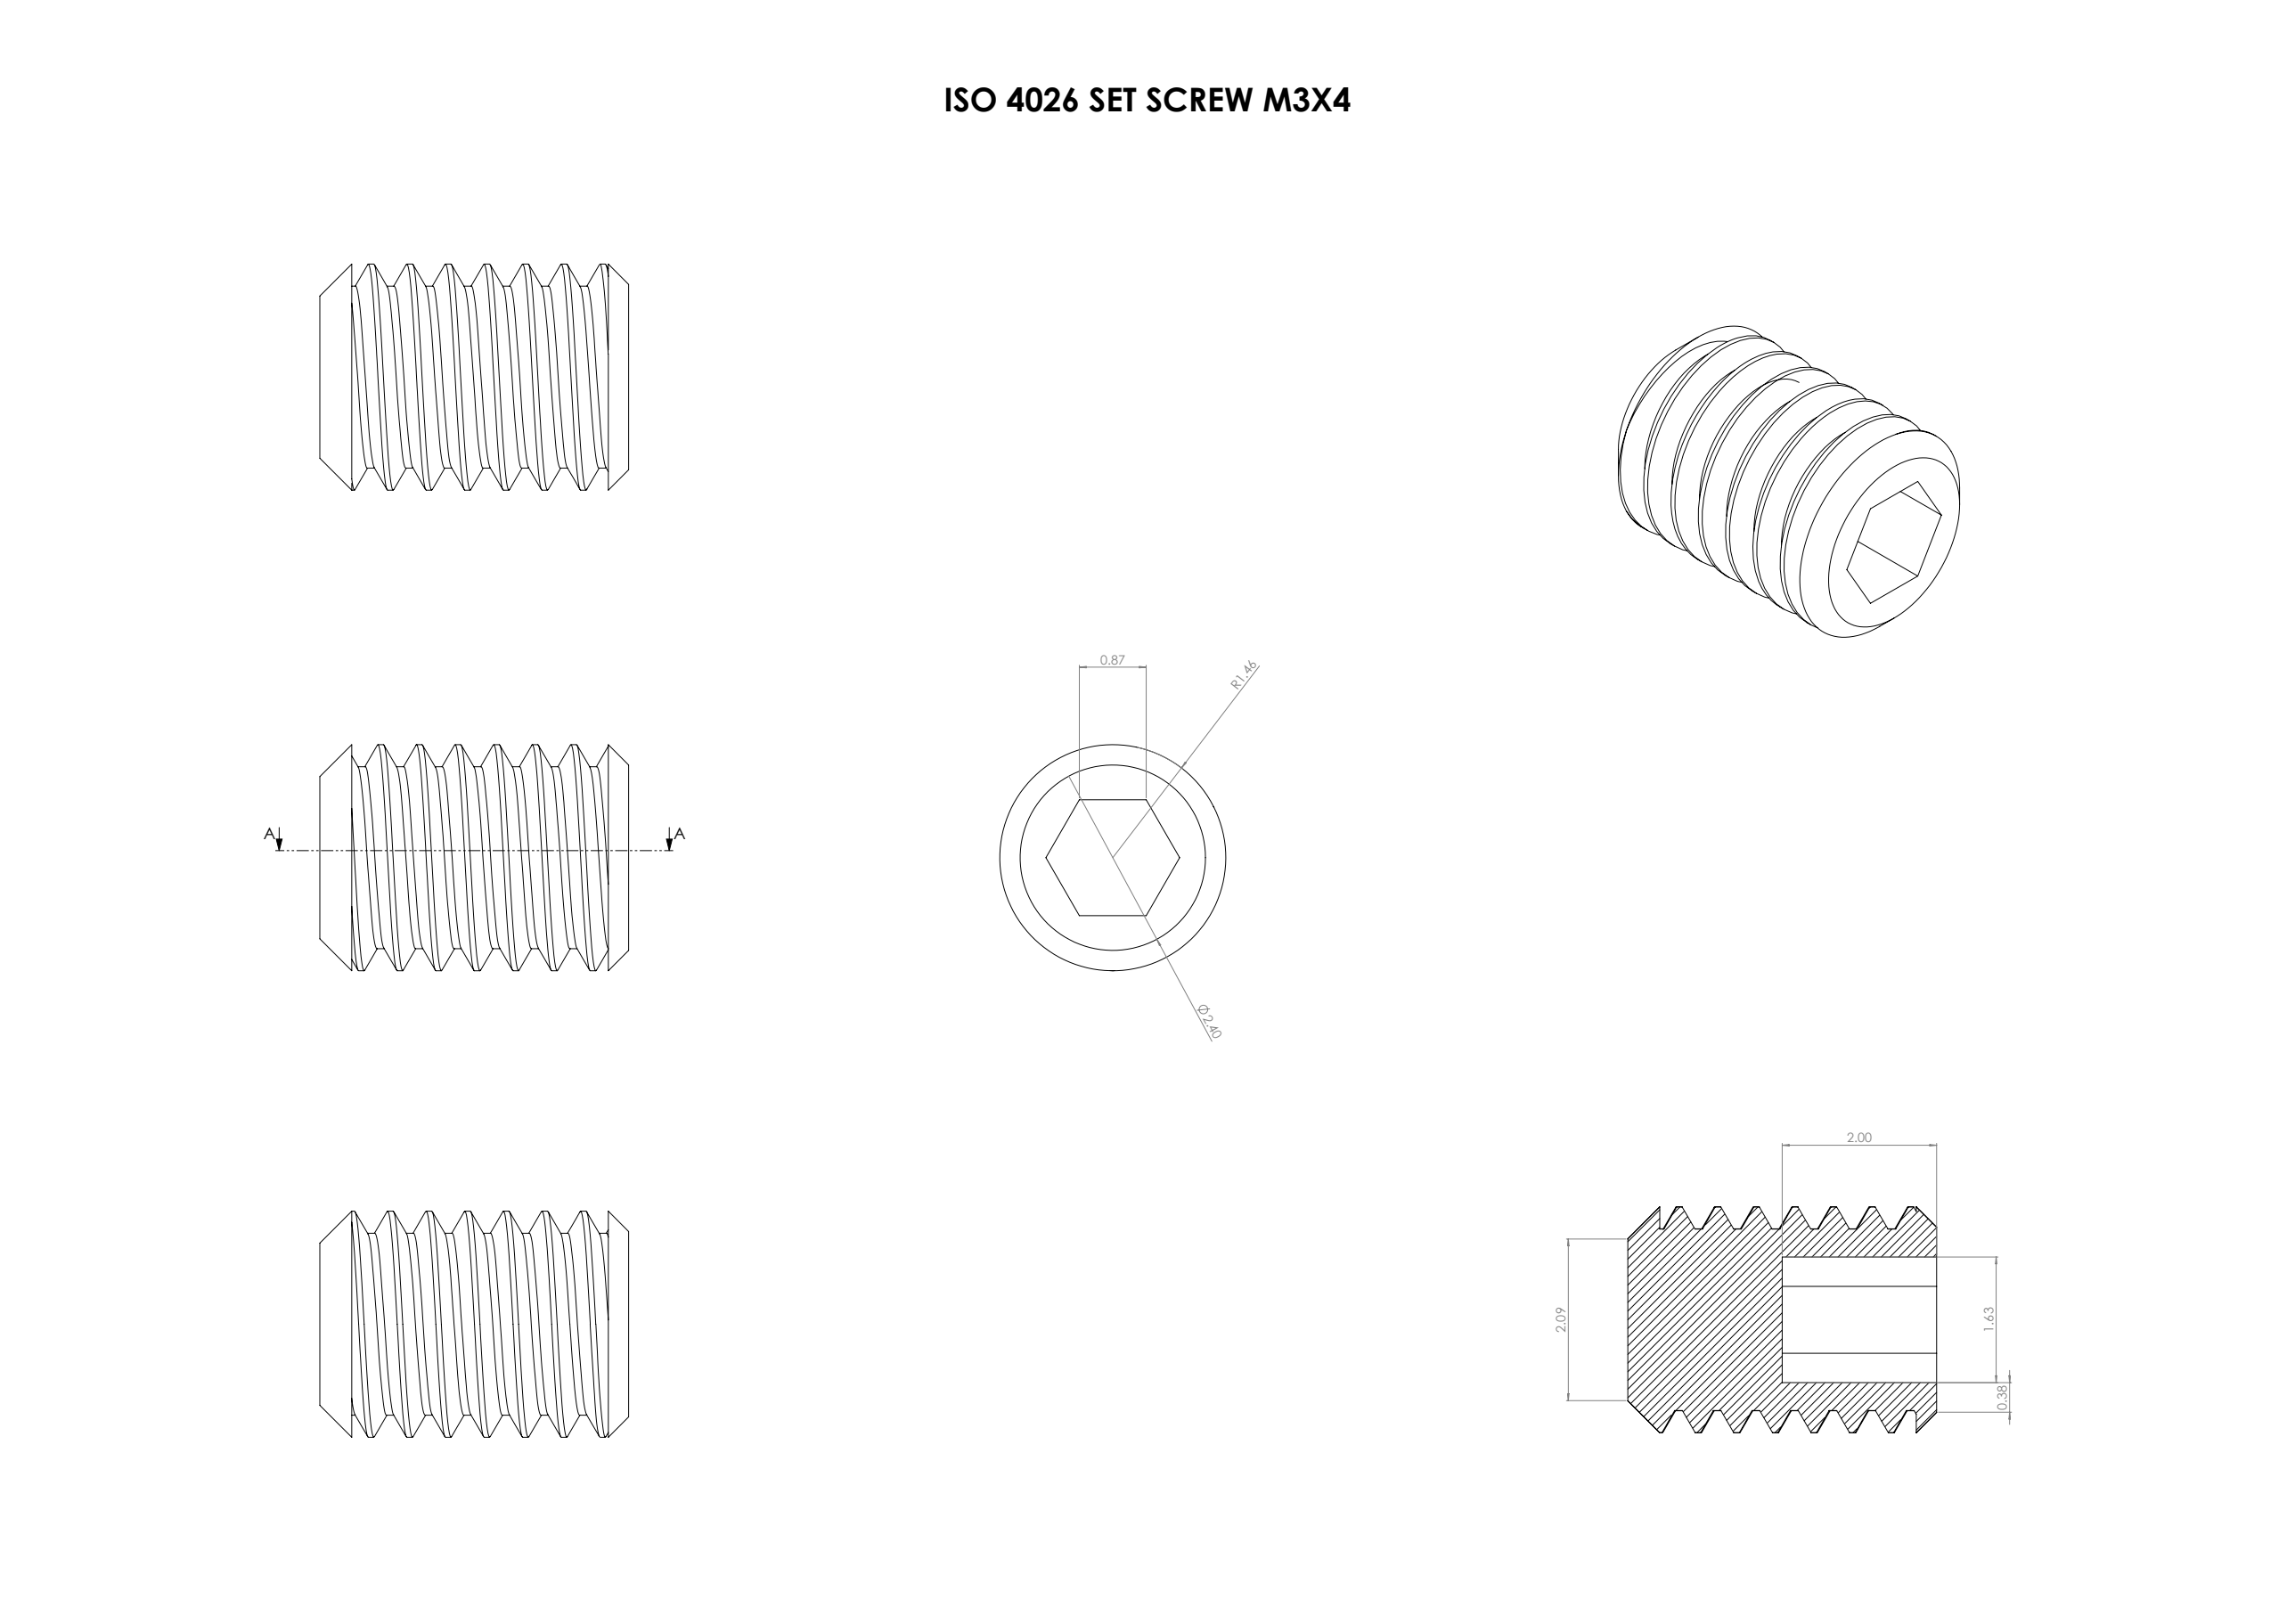
ISO-10303-21;
HEADER;
/* Generated by software containing ST-Developer
 * from STEP Tools, Inc. (www.steptools.com) 
 */

FILE_DESCRIPTION(
/* description */ (''),
/* implementation_level */ '2;1');

FILE_NAME(
/* name */ '19_ISO_4026_Set_Screw_M3x4.step',
/* time_stamp */ '2026-10-21T01:56:51-07:00',
/* author */ (''),
/* organization */ (''),
/* preprocessor_version */ 'ST-DEVELOPER v20.2',
/* originating_system */ 'Autodesk Translation Framework v15.15.0.0',
/* authorisation */ '');

FILE_SCHEMA (('AUTOMOTIVE_DESIGN { 1 0 10303 214 3 1 1 }'));
ENDSEC;

DATA;
#10=MECHANICAL_DESIGN_GEOMETRIC_PRESENTATION_REPRESENTATION('',(#288),#82384);
#250=SHAPE_REPRESENTATION_RELATIONSHIP('SRR','None',#82484,#269);
#269=ADVANCED_BREP_SHAPE_REPRESENTATION('',(#307),#82383);
#288=STYLED_ITEM('',(#82638),#307);
#307=MANIFOLD_SOLID_BREP('Body1',#30679);
#431=B_SPLINE_SURFACE_WITH_KNOTS('',3,3,((#81664,#81665,#81666,#81667,#81668,
#81669,#81670,#81671,#81672,#81673,#81674,#81675,#81676,#81677,#81678,#81679,
#81680,#81681,#81682,#81683,#81684,#81685,#81686,#81687,#81688,#81689,#81690,
#81691,#81692,#81693,#81694,#81695,#81696,#81697,#81698,#81699,#81700,#81701,
#81702,#81703,#81704,#81705,#81706,#81707,#81708,#81709,#81710),(#81711,
#81712,#81713,#81714,#81715,#81716,#81717,#81718,#81719,#81720,#81721,#81722,
#81723,#81724,#81725,#81726,#81727,#81728,#81729,#81730,#81731,#81732,#81733,
#81734,#81735,#81736,#81737,#81738,#81739,#81740,#81741,#81742,#81743,#81744,
#81745,#81746,#81747,#81748,#81749,#81750,#81751,#81752,#81753,#81754,#81755,
#81756,#81757),(#81758,#81759,#81760,#81761,#81762,#81763,#81764,#81765,
#81766,#81767,#81768,#81769,#81770,#81771,#81772,#81773,#81774,#81775,#81776,
#81777,#81778,#81779,#81780,#81781,#81782,#81783,#81784,#81785,#81786,#81787,
#81788,#81789,#81790,#81791,#81792,#81793,#81794,#81795,#81796,#81797,#81798,
#81799,#81800,#81801,#81802,#81803,#81804),(#81805,#81806,#81807,#81808,
#81809,#81810,#81811,#81812,#81813,#81814,#81815,#81816,#81817,#81818,#81819,
#81820,#81821,#81822,#81823,#81824,#81825,#81826,#81827,#81828,#81829,#81830,
#81831,#81832,#81833,#81834,#81835,#81836,#81837,#81838,#81839,#81840,#81841,
#81842,#81843,#81844,#81845,#81846,#81847,#81848,#81849,#81850,#81851)),
 .UNSPECIFIED.,.F.,.F.,.F.,(4,4),(4,1,1,1,1,1,1,1,1,1,1,1,1,1,1,1,1,1,1,
1,1,1,1,1,1,1,1,1,1,1,1,1,1,1,1,1,1,1,1,1,1,1,1,1,4),(0.,0.0329955678841871),
(8.30203615430838,9.29820029578191,10.2943644372554,11.290528578729,12.2866927202025,
13.282856861676,14.2790210031496,15.2751851446231,16.2713492860966,17.2675134275701,
18.2636775690437,19.2598417105172,20.2560058519907,21.2521699934642,22.2483341349378,
23.2444982764113,24.2406624178848,25.2368265593584,26.2329907008319,27.2291548423054,
28.225318983779,29.2214831252525,30.217647266726,31.2138114081995,32.2099755496731,
33.2061396911466,34.2023038326201,35.1984679740937,36.1946321155672,37.1907962570407,
38.1869603985142,39.1831245399878,40.1792886814613,41.1754528229348,42.1716169644084,
43.1677811058819,44.1639452473554,45.1601093888289,46.1562735303025,47.152437671776,
48.1486018132495,49.1447659547231,50.1409300961966,51.1370942376701,52.1332583791436),
 .UNSPECIFIED.);
#432=B_SPLINE_SURFACE_WITH_KNOTS('',3,3,((#82060,#82061,#82062,#82063,#82064,
#82065,#82066,#82067,#82068,#82069,#82070,#82071,#82072,#82073,#82074,#82075,
#82076,#82077,#82078,#82079,#82080,#82081,#82082,#82083,#82084,#82085,#82086,
#82087,#82088,#82089,#82090,#82091,#82092,#82093,#82094,#82095,#82096,#82097,
#82098,#82099,#82100,#82101,#82102,#82103,#82104,#82105,#82106),(#82107,
#82108,#82109,#82110,#82111,#82112,#82113,#82114,#82115,#82116,#82117,#82118,
#82119,#82120,#82121,#82122,#82123,#82124,#82125,#82126,#82127,#82128,#82129,
#82130,#82131,#82132,#82133,#82134,#82135,#82136,#82137,#82138,#82139,#82140,
#82141,#82142,#82143,#82144,#82145,#82146,#82147,#82148,#82149,#82150,#82151,
#82152,#82153),(#82154,#82155,#82156,#82157,#82158,#82159,#82160,#82161,
#82162,#82163,#82164,#82165,#82166,#82167,#82168,#82169,#82170,#82171,#82172,
#82173,#82174,#82175,#82176,#82177,#82178,#82179,#82180,#82181,#82182,#82183,
#82184,#82185,#82186,#82187,#82188,#82189,#82190,#82191,#82192,#82193,#82194,
#82195,#82196,#82197,#82198,#82199,#82200),(#82201,#82202,#82203,#82204,
#82205,#82206,#82207,#82208,#82209,#82210,#82211,#82212,#82213,#82214,#82215,
#82216,#82217,#82218,#82219,#82220,#82221,#82222,#82223,#82224,#82225,#82226,
#82227,#82228,#82229,#82230,#82231,#82232,#82233,#82234,#82235,#82236,#82237,
#82238,#82239,#82240,#82241,#82242,#82243,#82244,#82245,#82246,#82247)),
 .UNSPECIFIED.,.F.,.F.,.F.,(4,4),(4,1,1,1,1,1,1,1,1,1,1,1,1,1,1,1,1,1,1,
1,1,1,1,1,1,1,1,1,1,1,1,1,1,1,1,1,1,1,1,1,1,1,1,1,4),(0.,0.0329955678841871),
(11.6159397475004,12.6121038889739,13.6082680304475,14.604432171921,15.6005963133945,
16.5967604548681,17.5929245963416,18.5890887378151,19.5852528792886,20.5814170207622,
21.5775811622357,22.5737453037092,23.5699094451828,24.5660735866563,25.5622377281298,
26.5584018696034,27.5545660110769,28.5507301525504,29.5468942940239,30.5430584354975,
31.539222576971,32.5353867184445,33.531550859918,34.5277150013916,35.5238791428651,
36.5200432843386,37.5162074258122,38.5123715672857,39.5085357087592,40.5046998502328,
41.5008639917063,42.4970281331798,43.4931922746533,44.4893564161269,45.4855205576004,
46.4816846990739,47.4778488405475,48.474012982021,49.4701771234945,50.466341264968,
51.4625054064416,52.4586695479151,53.4548336893886,54.4509978308621,55.4471619723357),
 .UNSPECIFIED.);
#1021=CYLINDRICAL_SURFACE('',#33339,1.4635);
#1022=CYLINDRICAL_SURFACE('',#33341,1.4635);
#1023=CYLINDRICAL_SURFACE('',#33342,1.4635);
#1024=CYLINDRICAL_SURFACE('',#33343,1.4635);
#1025=CYLINDRICAL_SURFACE('',#33344,1.4635);
#1026=CYLINDRICAL_SURFACE('',#33345,1.4635);
#1027=CYLINDRICAL_SURFACE('',#33346,1.4635);
#1028=CYLINDRICAL_SURFACE('',#33347,1.17775);
#1029=CYLINDRICAL_SURFACE('',#33349,1.17775);
#1030=CYLINDRICAL_SURFACE('',#33350,1.17775);
#1031=CYLINDRICAL_SURFACE('',#33351,1.17775);
#1032=CYLINDRICAL_SURFACE('',#33352,1.17775);
#1033=CYLINDRICAL_SURFACE('',#33353,1.17775);
#1034=CYLINDRICAL_SURFACE('',#33361,1.17775);
#1035=CYLINDRICAL_SURFACE('',#33372,1.4635);
#1862=CIRCLE('',#33340,1.4635);
#1863=CIRCLE('',#33348,1.17775);
#1864=CIRCLE('',#33355,1.4635);
#1865=CIRCLE('',#33356,1.4635);
#1866=CIRCLE('',#33358,1.4635);
#1867=CIRCLE('',#33359,1.4635);
#1868=CIRCLE('',#33360,1.17775);
#1869=CIRCLE('',#33370,1.05);
#1870=CIRCLE('',#33373,1.4635);
#1871=CIRCLE('',#33375,1.2);
#2081=CONICAL_SURFACE('',#33371,1.275,0.785398163397448);
#2082=CONICAL_SURFACE('',#33374,1.35,0.785398163397448);
#3250=B_SPLINE_CURVE_WITH_KNOTS('',3,(#81027,#81028,#81029,#81030,#81031,
#81032,#81033,#81034,#81035,#81036),.UNSPECIFIED.,.F.,.F.,(4,3,3,4),(-4.09202352044853,
-3.98465656589411,-2.98849242442058,-2.07317267331971),.UNSPECIFIED.);
#3251=B_SPLINE_CURVE_WITH_KNOTS('',3,(#81039,#81040,#81041,#81042,#81043,
#81044,#81045),.UNSPECIFIED.,.F.,.F.,(4,3,4),(0.,0.99616414147353,1.12274180646097),
 .UNSPECIFIED.);
#3252=B_SPLINE_CURVE_WITH_KNOTS('',3,(#81050,#81051,#81052,#81053,#81054,
#81055,#81056,#81057,#81058,#81059,#81060,#81061,#81062,#81063,#81064,#81065,
#81066,#81067,#81068,#81069,#81070,#81071),.UNSPECIFIED.,.F.,.F.,(4,3,3,
3,3,3,3,4),(-10.3752088276281,-9.96164141473529,-8.96547727326176,-7.96931313178823,
-6.9731489903147,-5.97698484884117,-4.98082070736764,-4.09202352044853),
 .UNSPECIFIED.);
#3253=B_SPLINE_CURVE_WITH_KNOTS('',3,(#81072,#81073,#81074,#81075,#81076,
#81077,#81078,#81079,#81080,#81081,#81082,#81083,#81084,#81085,#81086,#81087,
#81088,#81089,#81090,#81091,#81092,#81093),.UNSPECIFIED.,.F.,.F.,(4,3,3,
3,3,3,3,4),(1.12274180646097,1.99232828294706,2.98849242442059,3.98465656589411,
4.98082070736764,5.97698484884117,6.9731489903147,7.40592711364056),
 .UNSPECIFIED.);
#3254=B_SPLINE_CURVE_WITH_KNOTS('',3,(#81098,#81099,#81100,#81101,#81102,
#81103,#81104,#81105,#81106,#81107,#81108,#81109,#81110,#81111,#81112,#81113,
#81114,#81115,#81116,#81117,#81118,#81119),.UNSPECIFIED.,.F.,.F.,(4,3,3,
3,3,3,3,4),(-16.6583941348077,-15.9386262635765,-14.9424621221029,-13.9462979806294,
-12.9501338391559,-11.9539696976823,-10.9578055562088,-10.3752088276281),
 .UNSPECIFIED.);
#3255=B_SPLINE_CURVE_WITH_KNOTS('',3,(#81120,#81121,#81122,#81123,#81124,
#81125,#81126,#81127,#81128,#81129,#81130,#81131,#81132,#81133,#81134,#81135,
#81136,#81137,#81138,#81139,#81140,#81141),.UNSPECIFIED.,.F.,.F.,(4,3,3,
3,3,3,3,4),(7.40592711364056,7.96931313178823,8.96547727326176,9.96164141473529,
10.9578055562088,11.9539696976823,12.9501338391559,13.6891124208201),
 .UNSPECIFIED.);
#3256=B_SPLINE_CURVE_WITH_KNOTS('',3,(#81146,#81147,#81148,#81149,#81150,
#81151,#81152,#81153,#81154,#81155,#81156,#81157,#81158,#81159,#81160,#81161,
#81162,#81163,#81164,#81165,#81166,#81167,#81168,#81169,#81170),
 .UNSPECIFIED.,.F.,.F.,(4,3,3,3,3,3,3,3,4),(-22.9415794419873,-22.9117752538912,
-21.9156111124176,-20.9194469709441,-19.9232828294706,-18.927118687997,
-17.9309545465235,-16.93479040505,-16.6583941348077),.UNSPECIFIED.);
#3257=B_SPLINE_CURVE_WITH_KNOTS('',3,(#81171,#81172,#81173,#81174,#81175,
#81176,#81177,#81178,#81179,#81180,#81181,#81182,#81183,#81184,#81185,#81186,
#81187,#81188,#81189,#81190,#81191,#81192,#81193,#81194,#81195),
 .UNSPECIFIED.,.F.,.F.,(4,3,3,3,3,3,3,3,4),(13.6891124208201,13.9462979806294,
14.9424621221029,15.9386262635765,16.93479040505,17.9309545465235,18.927118687997,
19.9232828294706,19.9722977279997),.UNSPECIFIED.);
#3258=B_SPLINE_CURVE_WITH_KNOTS('',3,(#81200,#81201,#81202,#81203,#81204,
#81205,#81206,#81207,#81208,#81209,#81210,#81211,#81212,#81213,#81214,#81215,
#81216,#81217,#81218,#81219,#81220,#81221),.UNSPECIFIED.,.F.,.F.,(4,3,3,
3,3,3,3,4),(-29.2247647491669,-28.8887601027323,-27.8925959612588,-26.8964318197853,
-25.9002676783117,-24.9041035368382,-23.9079393953647,-22.9415794419873),
 .UNSPECIFIED.);
#3259=B_SPLINE_CURVE_WITH_KNOTS('',3,(#81222,#81223,#81224,#81225,#81226,
#81227,#81228,#81229,#81230,#81231,#81232,#81233,#81234,#81235,#81236,#81237,
#81238,#81239,#81240,#81241,#81242,#81243),.UNSPECIFIED.,.F.,.F.,(4,3,3,
3,3,3,3,4),(19.9722977279997,20.9194469709441,21.9156111124176,22.9117752538912,
23.9079393953647,24.9041035368382,25.9002676783117,26.2554830351793),
 .UNSPECIFIED.);
#3260=B_SPLINE_CURVE_WITH_KNOTS('',3,(#81248,#81249,#81250,#81251,#81252,
#81253,#81254,#81255,#81256,#81257,#81258,#81259,#81260,#81261,#81262,#81263,
#81264,#81265,#81266,#81267,#81268,#81269),.UNSPECIFIED.,.F.,.F.,(4,3,3,
3,3,3,3,4),(-35.5079500563465,-34.8657449515735,-33.8695808101,-32.8734166686264,
-31.8772525271529,-30.8810883856794,-29.8849242442059,-29.2247647491669),
 .UNSPECIFIED.);
#3261=B_SPLINE_CURVE_WITH_KNOTS('',3,(#81270,#81271,#81272,#81273,#81274,
#81275,#81276,#81277,#81278,#81279,#81280,#81281,#81282,#81283,#81284,#81285,
#81286,#81287,#81288,#81289,#81290,#81291),.UNSPECIFIED.,.F.,.F.,(4,3,3,
3,3,3,3,4),(26.2554830351793,26.8964318197853,27.8925959612588,28.8887601027323,
29.8849242442059,30.8810883856794,31.8772525271529,32.5386683423589),
 .UNSPECIFIED.);
#3262=B_SPLINE_CURVE_WITH_KNOTS('',3,(#81296,#81297,#81298,#81299,#81300,
#81301,#81302,#81303,#81304,#81305,#81306,#81307,#81308,#81309,#81310,#81311,
#81312,#81313,#81314,#81315,#81316,#81317),.UNSPECIFIED.,.F.,.F.,(4,3,3,
3,3,3,3,4),(-41.791135363526,-40.8427298004147,-39.8465656589411,-38.8504015174676,
-37.8542373759941,-36.8580732345206,-35.861909093047,-35.5079500563465),
 .UNSPECIFIED.);
#3263=B_SPLINE_CURVE_WITH_KNOTS('',3,(#81318,#81319,#81320,#81321,#81322,
#81323,#81324,#81325,#81326,#81327,#81328,#81329,#81330,#81331,#81332,#81333,
#81334,#81335,#81336,#81337,#81338,#81339),.UNSPECIFIED.,.F.,.F.,(4,3,3,
3,3,3,3,4),(32.5386683423589,32.8734166686265,33.8695808101,34.8657449515735,
35.861909093047,36.8580732345206,37.8542373759941,38.8218536495385),
 .UNSPECIFIED.);
#3264=B_SPLINE_CURVE_WITH_KNOTS('',3,(#81345,#81346,#81347,#81348,#81349,
#81350,#81351,#81352,#81353,#81354),.UNSPECIFIED.,.F.,.F.,(4,1,1,1,1,1,
1,4),(47.1238898038469,47.4778488405475,48.474012982021,49.4701771234945,
50.466341264968,51.4625054064416,52.4586695479151,53.373989299016),
 .UNSPECIFIED.);
#3265=B_SPLINE_CURVE_WITH_KNOTS('',3,(#81357,#81358,#81359,#81360,#81361,
#81362,#81363,#81364,#81365),.UNSPECIFIED.,.F.,.F.,(4,1,1,1,1,1,4),(47.1238898038469,
47.152437671776,48.1486018132495,49.1447659547231,50.1409300961966,51.1370942376701,
52.1332583791436),.UNSPECIFIED.);
#3266=B_SPLINE_CURVE_WITH_KNOTS('',3,(#81370,#81371,#81372,#81373,#81374,
#81375,#81376,#81377,#81378,#81379),.UNSPECIFIED.,.F.,.F.,(4,1,1,1,1,1,
1,4),(40.8407044966673,41.5008639917063,42.4970281331798,43.4931922746533,
44.4893564161269,45.4855205576004,46.4816846990739,47.1238898038469),
 .UNSPECIFIED.);
#3267=B_SPLINE_CURVE_WITH_KNOTS('',3,(#81380,#81381,#81382,#81383,#81384,
#81385,#81386,#81387,#81388,#81389),.UNSPECIFIED.,.F.,.F.,(4,1,1,1,1,1,
1,4),(40.8407044966673,41.1754528229348,42.1716169644084,43.1677811058819,
44.1639452473554,45.1601093888289,46.1562735303025,47.1238898038469),
 .UNSPECIFIED.);
#3268=B_SPLINE_CURVE_WITH_KNOTS('',3,(#81394,#81395,#81396,#81397,#81398,
#81399,#81400,#81401,#81402,#81403),.UNSPECIFIED.,.F.,.F.,(4,1,1,1,1,1,
1,4),(34.5575191894877,35.5238791428651,36.5200432843386,37.5162074258122,
38.5123715672857,39.5085357087592,40.5046998502328,40.8407044966673),
 .UNSPECIFIED.);
#3269=B_SPLINE_CURVE_WITH_KNOTS('',3,(#81404,#81405,#81406,#81407,#81408,
#81409,#81410,#81411,#81412,#81413),.UNSPECIFIED.,.F.,.F.,(4,1,1,1,1,1,
1,4),(34.5575191894877,35.1984679740937,36.1946321155672,37.1907962570407,
38.1869603985142,39.1831245399878,40.1792886814613,40.8407044966673),
 .UNSPECIFIED.);
#3270=B_SPLINE_CURVE_WITH_KNOTS('',3,(#81418,#81419,#81420,#81421,#81422,
#81423,#81424,#81425,#81426,#81427,#81428),.UNSPECIFIED.,.F.,.F.,(4,1,1,
1,1,1,1,1,4),(28.2743338823081,28.5507301525504,29.5468942940239,30.5430584354975,
31.539222576971,32.5353867184445,33.531550859918,34.5277150013916,34.5575191894877),
 .UNSPECIFIED.);
#3271=B_SPLINE_CURVE_WITH_KNOTS('',3,(#81429,#81430,#81431,#81432,#81433,
#81434,#81435,#81436,#81437,#81438),.UNSPECIFIED.,.F.,.F.,(4,1,1,1,1,1,
1,4),(28.2743338823081,29.2214831252525,30.217647266726,31.2138114081995,
32.2099755496731,33.2061396911466,34.2023038326201,34.5575191894877),
 .UNSPECIFIED.);
#3272=B_SPLINE_CURVE_WITH_KNOTS('',3,(#81443,#81444,#81445,#81446,#81447,
#81448,#81449,#81450,#81451,#81452),.UNSPECIFIED.,.F.,.F.,(4,1,1,1,1,1,
1,4),(21.9911485751285,22.5737453037092,23.5699094451828,24.5660735866563,
25.5622377281298,26.5584018696034,27.5545660110769,28.2743338823081),
 .UNSPECIFIED.);
#3273=B_SPLINE_CURVE_WITH_KNOTS('',3,(#81453,#81454,#81455,#81456,#81457,
#81458,#81459,#81460,#81461,#81462,#81463),.UNSPECIFIED.,.F.,.F.,(4,1,1,
1,1,1,1,1,4),(21.9911485751285,22.2483341349378,23.2444982764113,24.2406624178848,
25.2368265593584,26.2329907008319,27.2291548423054,28.225318983779,28.2743338823081),
 .UNSPECIFIED.);
#3274=B_SPLINE_CURVE_WITH_KNOTS('',3,(#81468,#81469,#81470,#81471,#81472,
#81473,#81474,#81475,#81476,#81477),.UNSPECIFIED.,.F.,.F.,(4,1,1,1,1,1,
1,4),(15.707963267949,16.5967604548681,17.5929245963416,18.5890887378151,
19.5852528792886,20.5814170207622,21.5775811622357,21.9911485751285),
 .UNSPECIFIED.);
#3275=B_SPLINE_CURVE_WITH_KNOTS('',3,(#81478,#81479,#81480,#81481,#81482,
#81483,#81484,#81485,#81486,#81487),.UNSPECIFIED.,.F.,.F.,(4,1,1,1,1,1,
1,4),(15.7079632679489,16.2713492860966,17.2675134275701,18.2636775690437,
19.2598417105172,20.2560058519907,21.2521699934642,21.9911485751285),
 .UNSPECIFIED.);
#3276=B_SPLINE_CURVE_WITH_KNOTS('',3,(#81490,#81491,#81492,#81493,#81494,
#81495,#81496,#81497,#81498,#81499,#81500,#81501,#81502,#81503,#81504,#81505,
#81506,#81507,#81508,#81509,#81510,#81511,#81512,#81513,#81514,#81515,#81516,
#81517,#81518,#81519,#81520,#81521,#81522,#81523,#81524,#81525,#81526,#81527,
#81528,#81529,#81530,#81531,#81532,#81533,#81534,#81535,#81536,#81537,#81538,
#81539,#81540,#81541,#81542,#81543,#81544,#81545,#81546,#81547,#81548,#81549,
#81550,#81551,#81552,#81553,#81554,#81555,#81556,#81557,#81558,#81559,#81560,
#81561,#81562,#81563,#81564,#81565,#81566,#81567,#81568,#81569,#81570,#81571,
#81572,#81573,#81574),.UNSPECIFIED.,.F.,.F.,(4,3,3,3,3,3,3,3,3,3,3,3,3,
3,3,3,3,3,3,3,3,3,3,3,3,3,3,3,4),(-0.276631791712725,-0.266952028164814,
-0.252323120380107,-0.245291696267628,-0.242250024468316,-0.226984993323628,
-0.216140129019276,-0.211926830943687,-0.208887036385599,-0.193126552069373,
-0.177076639522004,-0.167863999363706,-0.162681055949887,-0.159693750396033,
-0.143166615227965,-0.140226078888815,-0.124274134827967,-0.116088608730203,
-0.111105706457781,-0.107817001525543,-0.0912655983034208,-0.0743533570119642,
-0.0648492915702117,-0.0586243521231257,-0.055485434306559,-0.0380411261163856,
-0.0205521325003434,-0.00346624990959772,0.),.UNSPECIFIED.);
#3277=B_SPLINE_CURVE_WITH_KNOTS('',3,(#81579,#81580,#81581,#81582,#81583,
#81584,#81585,#81586,#81587,#81588,#81589,#81590,#81591,#81592,#81593,#81594,
#81595,#81596,#81597,#81598,#81599,#81600,#81601,#81602,#81603,#81604,#81605,
#81606,#81607,#81608,#81609,#81610,#81611,#81612,#81613,#81614,#81615,#81616,
#81617,#81618,#81619,#81620,#81621,#81622,#81623,#81624,#81625,#81626,#81627,
#81628,#81629,#81630,#81631,#81632,#81633,#81634,#81635,#81636,#81637,#81638,
#81639,#81640,#81641,#81642,#81643,#81644,#81645,#81646,#81647,#81648,#81649,
#81650,#81651,#81652,#81653,#81654,#81655,#81656,#81657,#81658,#81659,#81660,
#81661,#81662,#81663),.UNSPECIFIED.,.F.,.F.,(4,3,3,3,3,3,3,3,3,3,3,3,3,
3,3,3,3,3,3,3,3,3,3,3,3,3,3,3,4),(-0.275362278356886,-0.263558129214759,
-0.246259601438028,-0.240454824668648,-0.236894340710815,-0.233127676432609,
-0.215926618879135,-0.204582029894356,-0.20054686414582,-0.196717291630079,
-0.179965358204731,-0.163633434810385,-0.154017552858015,-0.14710518062374,
-0.144181207184443,-0.128328561127056,-0.125169907000906,-0.10816649509411,
-0.10086959066255,-0.0956369517540662,-0.0926001968852286,-0.0768321091103029,
-0.0611424409132595,-0.0532927242788775,-0.0475055755195517,-0.0447074663570426,
-0.0295993711118811,-0.0147996855559406,0.),.UNSPECIFIED.);
#3278=B_SPLINE_CURVE_WITH_KNOTS('',3,(#81852,#81853,#81854,#81855,#81856,
#81857,#81858,#81859,#81860,#81861,#81862,#81863,#81864),.UNSPECIFIED.,
 .F.,.F.,(4,3,3,3,4),(38.8218536495385,38.8504015174676,39.8465656589411,
40.8427298004147,41.7580495515155),.UNSPECIFIED.);
#3279=B_SPLINE_CURVE_WITH_KNOTS('',3,(#81866,#81867,#81868,#81869,#81870,
#81871,#81872,#81873,#81874,#81875,#81876,#81877,#81878,#81879,#81880,#81881,
#81882,#81883,#81884,#81885,#81886,#81887,#81888,#81889,#81890,#81891,#81892,
#81893,#81894,#81895,#81896,#81897,#81898,#81899,#81900,#81901,#81902,#81903,
#81904,#81905,#81906,#81907,#81908,#81909,#81910,#81911,#81912,#81913,#81914,
#81915,#81916,#81917,#81918,#81919,#81920,#81921,#81922,#81923,#81924,#81925,
#81926,#81927,#81928,#81929,#81930,#81931,#81932,#81933,#81934,#81935,#81936,
#81937,#81938,#81939,#81940,#81941,#81942,#81943,#81944,#81945,#81946,#81947,
#81948,#81949,#81950),.UNSPECIFIED.,.F.,.F.,(4,3,3,3,3,3,3,3,3,3,3,3,3,
3,3,3,3,3,3,3,3,3,3,3,3,3,3,3,4),(-0.276631791712723,-0.266952028164814,
-0.252323110100293,-0.245291653864685,-0.242249974245191,-0.226984934997862,
-0.216140077984231,-0.211926799186654,-0.208886967893919,-0.193126476631429,
-0.177076564913133,-0.167863943407054,-0.162681030994628,-0.159693742323349,
-0.143166607617838,-0.140226078888816,-0.124274130962391,-0.11608860686451,
-0.111105706623904,-0.10781700186492,-0.0912655940336371,-0.0743533484091529,
-0.0648492894661215,-0.0586243472175359,-0.0554854283171653,-0.0380411167797804,
-0.020552125725747,-0.00346625662044922,0.),.UNSPECIFIED.);
#3280=B_SPLINE_CURVE_WITH_KNOTS('',3,(#81951,#81952,#81953,#81954,#81955,
#81956,#81957,#81958,#81959),.UNSPECIFIED.,.F.,.F.,(4,1,1,1,1,1,4),(10.3752088276281,
11.290528578729,12.2866927202025,13.282856861676,14.2790210031496,15.2751851446231,
15.7079632679489),.UNSPECIFIED.);
#3281=B_SPLINE_CURVE_WITH_KNOTS('',3,(#81965,#81966,#81967,#81968,#81969,
#81970,#81971,#81972,#81973,#81974,#81975,#81976,#81977,#81978,#81979,#81980,
#81981,#81982,#81983,#81984,#81985,#81986,#81987,#81988,#81989,#81990,#81991,
#81992,#81993,#81994,#81995,#81996,#81997,#81998,#81999,#82000,#82001,#82002,
#82003,#82004,#82005,#82006,#82007,#82008,#82009,#82010,#82011,#82012,#82013,
#82014,#82015,#82016,#82017,#82018,#82019,#82020,#82021,#82022,#82023,#82024,
#82025,#82026,#82027,#82028,#82029,#82030,#82031,#82032,#82033,#82034,#82035,
#82036,#82037,#82038,#82039,#82040,#82041,#82042,#82043,#82044,#82045,#82046,
#82047,#82048,#82049),.UNSPECIFIED.,.F.,.F.,(4,3,3,3,3,3,3,3,3,3,3,3,3,
3,3,3,3,3,3,3,3,3,3,3,3,3,3,3,4),(-0.275362278356885,-0.263558129214756,
-0.246259601438024,-0.240454828090957,-0.236894346107961,-0.233127679120847,
-0.215926621847007,-0.204582032491244,-0.200546888044474,-0.196717301354411,
-0.17996536893454,-0.163633454327148,-0.154017567495587,-0.147105232827191,
-0.144181241921046,-0.128328604154869,-0.125169907000904,-0.108166390597872,
-0.100869563000488,-0.0956369336203211,-0.0926001921206514,-0.0768321064508614,
-0.0611424315003572,-0.0532927214375046,-0.0475055703614835,-0.0447074615733897,
-0.0295993573058915,-0.0147996786529457,0.),.UNSPECIFIED.);
#3282=B_SPLINE_CURVE_WITH_KNOTS('',3,(#82052,#82053,#82054,#82055,#82056,
#82057,#82058,#82059),.UNSPECIFIED.,.F.,.F.,(4,1,1,1,1,4),(11.6159397475004,
12.6121038889739,13.6082680304475,14.604432171921,15.6005963133945,15.707963267949),
 .UNSPECIFIED.);
#3283=B_SPLINE_CURVE_WITH_KNOTS('',3,(#82248,#82249,#82250,#82251,#82252,
#82253,#82254,#82255,#82256,#82257),.UNSPECIFIED.,.F.,.F.,(4,3,3,4),(-43.8312222248353,
-42.8350580833617,-41.8388939418882,-41.791135363526),.UNSPECIFIED.);
#3576=FACE_BOUND('',#7381,.T.);
#5303=FACE_OUTER_BOUND('',#7351,.T.);
#5304=FACE_OUTER_BOUND('',#7352,.T.);
#5305=FACE_OUTER_BOUND('',#7353,.T.);
#5306=FACE_OUTER_BOUND('',#7354,.T.);
#5307=FACE_OUTER_BOUND('',#7355,.T.);
#5308=FACE_OUTER_BOUND('',#7356,.T.);
#5309=FACE_OUTER_BOUND('',#7357,.T.);
#5310=FACE_OUTER_BOUND('',#7358,.T.);
#5311=FACE_OUTER_BOUND('',#7359,.T.);
#5312=FACE_OUTER_BOUND('',#7360,.T.);
#5313=FACE_OUTER_BOUND('',#7361,.T.);
#5314=FACE_OUTER_BOUND('',#7362,.T.);
#5315=FACE_OUTER_BOUND('',#7363,.T.);
#5316=FACE_OUTER_BOUND('',#7364,.T.);
#5317=FACE_OUTER_BOUND('',#7365,.T.);
#5318=FACE_OUTER_BOUND('',#7366,.T.);
#5319=FACE_OUTER_BOUND('',#7367,.T.);
#5320=FACE_OUTER_BOUND('',#7368,.T.);
#5321=FACE_OUTER_BOUND('',#7369,.T.);
#5322=FACE_OUTER_BOUND('',#7370,.T.);
#5323=FACE_OUTER_BOUND('',#7371,.T.);
#5324=FACE_OUTER_BOUND('',#7372,.T.);
#5325=FACE_OUTER_BOUND('',#7373,.T.);
#5326=FACE_OUTER_BOUND('',#7374,.T.);
#5327=FACE_OUTER_BOUND('',#7375,.T.);
#5328=FACE_OUTER_BOUND('',#7376,.T.);
#5329=FACE_OUTER_BOUND('',#7377,.T.);
#5330=FACE_OUTER_BOUND('',#7378,.T.);
#5331=FACE_OUTER_BOUND('',#7379,.T.);
#5332=FACE_OUTER_BOUND('',#7380,.T.);
#7351=EDGE_LOOP('',(#27941,#27942,#27943,#27944));
#7352=EDGE_LOOP('',(#27945,#27946,#27947,#27948));
#7353=EDGE_LOOP('',(#27949,#27950,#27951,#27952));
#7354=EDGE_LOOP('',(#27953,#27954,#27955,#27956));
#7355=EDGE_LOOP('',(#27957,#27958,#27959,#27960));
#7356=EDGE_LOOP('',(#27961,#27962,#27963,#27964));
#7357=EDGE_LOOP('',(#27965,#27966,#27967,#27968));
#7358=EDGE_LOOP('',(#27969,#27970,#27971,#27972));
#7359=EDGE_LOOP('',(#27973,#27974,#27975,#27976));
#7360=EDGE_LOOP('',(#27977,#27978,#27979,#27980));
#7361=EDGE_LOOP('',(#27981,#27982,#27983,#27984));
#7362=EDGE_LOOP('',(#27985,#27986,#27987,#27988));
#7363=EDGE_LOOP('',(#27989,#27990,#27991,#27992));
#7364=EDGE_LOOP('',(#27993,#27994,#27995,#27996,#27997));
#7365=EDGE_LOOP('',(#27998,#27999,#28000,#28001,#28002,#28003,#28004,#28005,
#28006,#28007,#28008,#28009,#28010,#28011,#28012,#28013,#28014));
#7366=EDGE_LOOP('',(#28015,#28016,#28017,#28018,#28019));
#7367=EDGE_LOOP('',(#28020,#28021,#28022,#28023));
#7368=EDGE_LOOP('',(#28024,#28025,#28026,#28027,#28028,#28029,#28030,#28031,
#28032,#28033,#28034,#28035,#28036,#28037,#28038,#28039,#28040));
#7369=EDGE_LOOP('',(#28041,#28042,#28043,#28044));
#7370=EDGE_LOOP('',(#28045,#28046,#28047,#28048));
#7371=EDGE_LOOP('',(#28049,#28050,#28051,#28052));
#7372=EDGE_LOOP('',(#28053,#28054,#28055,#28056));
#7373=EDGE_LOOP('',(#28057,#28058,#28059,#28060));
#7374=EDGE_LOOP('',(#28061,#28062,#28063,#28064));
#7375=EDGE_LOOP('',(#28065,#28066,#28067,#28068,#28069,#28070));
#7376=EDGE_LOOP('',(#28071));
#7377=EDGE_LOOP('',(#28072,#28073,#28074,#28075,#28076,#28077));
#7378=EDGE_LOOP('',(#28078,#28079,#28080,#28081));
#7379=EDGE_LOOP('',(#28082,#28083,#28084,#28085,#28086,#28087));
#7380=EDGE_LOOP('',(#28088));
#7381=EDGE_LOOP('',(#28089,#28090,#28091,#28092,#28093,#28094));
#9655=LINE('',#81025,#11961);
#9656=LINE('',#81049,#11962);
#9657=LINE('',#81097,#11963);
#9658=LINE('',#81145,#11964);
#9659=LINE('',#81199,#11965);
#9660=LINE('',#81247,#11966);
#9661=LINE('',#81295,#11967);
#9662=LINE('',#81343,#11968);
#9663=LINE('',#81369,#11969);
#9664=LINE('',#81393,#11970);
#9665=LINE('',#81417,#11971);
#9666=LINE('',#81442,#11972);
#9667=LINE('',#81467,#11973);
#9668=LINE('',#82261,#11974);
#9669=LINE('',#82263,#11975);
#9670=LINE('',#82265,#11976);
#9671=LINE('',#82266,#11977);
#9672=LINE('',#82269,#11978);
#9673=LINE('',#82271,#11979);
#9674=LINE('',#82272,#11980);
#9675=LINE('',#82275,#11981);
#9676=LINE('',#82277,#11982);
#9677=LINE('',#82278,#11983);
#9678=LINE('',#82281,#11984);
#9679=LINE('',#82283,#11985);
#9680=LINE('',#82284,#11986);
#9681=LINE('',#82287,#11987);
#9682=LINE('',#82289,#11988);
#9683=LINE('',#82290,#11989);
#9684=LINE('',#82292,#11990);
#9685=LINE('',#82293,#11991);
#9686=LINE('',#82299,#11992);
#9687=LINE('',#82305,#11993);
#11961=VECTOR('',#40586,1.5);
#11962=VECTOR('',#40591,1.5);
#11963=VECTOR('',#40594,1.5);
#11964=VECTOR('',#40597,1.5);
#11965=VECTOR('',#40600,1.5);
#11966=VECTOR('',#40603,1.5);
#11967=VECTOR('',#40606,1.5);
#11968=VECTOR('',#40609,1.17775);
#11969=VECTOR('',#40614,1.17775);
#11970=VECTOR('',#40617,1.17775);
#11971=VECTOR('',#40620,1.17775);
#11972=VECTOR('',#40623,1.17775);
#11973=VECTOR('',#40626,1.17775);
#11974=VECTOR('',#40645,10.);
#11975=VECTOR('',#40646,10.);
#11976=VECTOR('',#40647,10.);
#11977=VECTOR('',#40648,10.);
#11978=VECTOR('',#40651,10.);
#11979=VECTOR('',#40652,10.);
#11980=VECTOR('',#40653,10.);
#11981=VECTOR('',#40656,10.);
#11982=VECTOR('',#40657,10.);
#11983=VECTOR('',#40658,10.);
#11984=VECTOR('',#40661,10.);
#11985=VECTOR('',#40662,10.);
#11986=VECTOR('',#40663,10.);
#11987=VECTOR('',#40666,10.);
#11988=VECTOR('',#40667,10.);
#11989=VECTOR('',#40668,10.);
#11990=VECTOR('',#40671,10.);
#11991=VECTOR('',#40672,10.);
#11992=VECTOR('',#40681,1.275);
#11993=VECTOR('',#40690,1.35);
#14806=VERTEX_POINT('',#81023);
#14807=VERTEX_POINT('',#81024);
#14808=VERTEX_POINT('',#81026);
#14809=VERTEX_POINT('',#81037);
#14810=VERTEX_POINT('',#81047);
#14811=VERTEX_POINT('',#81048);
#14812=VERTEX_POINT('',#81095);
#14813=VERTEX_POINT('',#81096);
#14814=VERTEX_POINT('',#81143);
#14815=VERTEX_POINT('',#81144);
#14816=VERTEX_POINT('',#81197);
#14817=VERTEX_POINT('',#81198);
#14818=VERTEX_POINT('',#81245);
#14819=VERTEX_POINT('',#81246);
#14820=VERTEX_POINT('',#81293);
#14821=VERTEX_POINT('',#81294);
#14822=VERTEX_POINT('',#81341);
#14823=VERTEX_POINT('',#81342);
#14824=VERTEX_POINT('',#81344);
#14825=VERTEX_POINT('',#81355);
#14826=VERTEX_POINT('',#81367);
#14827=VERTEX_POINT('',#81368);
#14828=VERTEX_POINT('',#81391);
#14829=VERTEX_POINT('',#81392);
#14830=VERTEX_POINT('',#81415);
#14831=VERTEX_POINT('',#81416);
#14832=VERTEX_POINT('',#81440);
#14833=VERTEX_POINT('',#81441);
#14834=VERTEX_POINT('',#81465);
#14835=VERTEX_POINT('',#81466);
#14836=VERTEX_POINT('',#81489);
#14837=VERTEX_POINT('',#81575);
#14838=VERTEX_POINT('',#81577);
#14839=VERTEX_POINT('',#81865);
#14840=VERTEX_POINT('',#81961);
#14841=VERTEX_POINT('',#81964);
#14842=VERTEX_POINT('',#82259);
#14843=VERTEX_POINT('',#82260);
#14844=VERTEX_POINT('',#82262);
#14845=VERTEX_POINT('',#82264);
#14846=VERTEX_POINT('',#82268);
#14847=VERTEX_POINT('',#82270);
#14848=VERTEX_POINT('',#82274);
#14849=VERTEX_POINT('',#82276);
#14850=VERTEX_POINT('',#82280);
#14851=VERTEX_POINT('',#82282);
#14852=VERTEX_POINT('',#82286);
#14853=VERTEX_POINT('',#82288);
#14854=VERTEX_POINT('',#82296);
#14855=VERTEX_POINT('',#82303);
#19192=EDGE_CURVE('',#14806,#14807,#9655,.T.);
#19193=EDGE_CURVE('',#14806,#14808,#3250,.T.);
#19194=EDGE_CURVE('',#14808,#14809,#1862,.T.);
#19195=EDGE_CURVE('',#14809,#14807,#3251,.T.);
#19196=EDGE_CURVE('',#14810,#14811,#9656,.T.);
#19197=EDGE_CURVE('',#14810,#14806,#3252,.T.);
#19198=EDGE_CURVE('',#14807,#14811,#3253,.T.);
#19199=EDGE_CURVE('',#14812,#14813,#9657,.T.);
#19200=EDGE_CURVE('',#14812,#14810,#3254,.T.);
#19201=EDGE_CURVE('',#14811,#14813,#3255,.T.);
#19202=EDGE_CURVE('',#14814,#14815,#9658,.T.);
#19203=EDGE_CURVE('',#14814,#14812,#3256,.T.);
#19204=EDGE_CURVE('',#14813,#14815,#3257,.T.);
#19205=EDGE_CURVE('',#14816,#14817,#9659,.T.);
#19206=EDGE_CURVE('',#14816,#14814,#3258,.T.);
#19207=EDGE_CURVE('',#14815,#14817,#3259,.T.);
#19208=EDGE_CURVE('',#14818,#14819,#9660,.T.);
#19209=EDGE_CURVE('',#14818,#14816,#3260,.T.);
#19210=EDGE_CURVE('',#14817,#14819,#3261,.T.);
#19211=EDGE_CURVE('',#14820,#14821,#9661,.T.);
#19212=EDGE_CURVE('',#14820,#14818,#3262,.T.);
#19213=EDGE_CURVE('',#14819,#14821,#3263,.T.);
#19214=EDGE_CURVE('',#14822,#14823,#9662,.T.);
#19215=EDGE_CURVE('',#14822,#14824,#3264,.T.);
#19216=EDGE_CURVE('',#14825,#14824,#1863,.T.);
#19217=EDGE_CURVE('',#14823,#14825,#3265,.T.);
#19218=EDGE_CURVE('',#14826,#14827,#9663,.T.);
#19219=EDGE_CURVE('',#14826,#14822,#3266,.T.);
#19220=EDGE_CURVE('',#14827,#14823,#3267,.T.);
#19221=EDGE_CURVE('',#14828,#14829,#9664,.T.);
#19222=EDGE_CURVE('',#14828,#14826,#3268,.T.);
#19223=EDGE_CURVE('',#14829,#14827,#3269,.T.);
#19224=EDGE_CURVE('',#14830,#14831,#9665,.T.);
#19225=EDGE_CURVE('',#14830,#14828,#3270,.T.);
#19226=EDGE_CURVE('',#14831,#14829,#3271,.T.);
#19227=EDGE_CURVE('',#14832,#14833,#9666,.T.);
#19228=EDGE_CURVE('',#14832,#14830,#3272,.T.);
#19229=EDGE_CURVE('',#14833,#14831,#3273,.T.);
#19230=EDGE_CURVE('',#14834,#14835,#9667,.T.);
#19231=EDGE_CURVE('',#14834,#14832,#3274,.T.);
#19232=EDGE_CURVE('',#14835,#14833,#3275,.T.);
#19233=EDGE_CURVE('',#14824,#14836,#3276,.T.);
#19234=EDGE_CURVE('',#14837,#14836,#1864,.F.);
#19235=EDGE_CURVE('',#14838,#14837,#1865,.F.);
#19236=EDGE_CURVE('',#14838,#14825,#3277,.T.);
#19237=EDGE_CURVE('',#14821,#14838,#3278,.T.);
#19238=EDGE_CURVE('',#14839,#14809,#3279,.T.);
#19239=EDGE_CURVE('',#14839,#14835,#3280,.T.);
#19240=EDGE_CURVE('',#14809,#14840,#1866,.T.);
#19241=EDGE_CURVE('',#14840,#14808,#1867,.T.);
#19242=EDGE_CURVE('',#14808,#14841,#3281,.T.);
#19243=EDGE_CURVE('',#14841,#14839,#1868,.T.);
#19244=EDGE_CURVE('',#14841,#14834,#3282,.T.);
#19245=EDGE_CURVE('',#14836,#14820,#3283,.T.);
#19246=EDGE_CURVE('',#14842,#14843,#9668,.T.);
#19247=EDGE_CURVE('',#14842,#14844,#9669,.T.);
#19248=EDGE_CURVE('',#14844,#14845,#9670,.T.);
#19249=EDGE_CURVE('',#14843,#14845,#9671,.T.);
#19250=EDGE_CURVE('',#14846,#14842,#9672,.T.);
#19251=EDGE_CURVE('',#14846,#14847,#9673,.T.);
#19252=EDGE_CURVE('',#14847,#14844,#9674,.T.);
#19253=EDGE_CURVE('',#14848,#14846,#9675,.T.);
#19254=EDGE_CURVE('',#14848,#14849,#9676,.T.);
#19255=EDGE_CURVE('',#14849,#14847,#9677,.T.);
#19256=EDGE_CURVE('',#14850,#14848,#9678,.T.);
#19257=EDGE_CURVE('',#14850,#14851,#9679,.T.);
#19258=EDGE_CURVE('',#14851,#14849,#9680,.T.);
#19259=EDGE_CURVE('',#14852,#14850,#9681,.T.);
#19260=EDGE_CURVE('',#14852,#14853,#9682,.T.);
#19261=EDGE_CURVE('',#14853,#14851,#9683,.T.);
#19262=EDGE_CURVE('',#14843,#14852,#9684,.T.);
#19263=EDGE_CURVE('',#14845,#14853,#9685,.T.);
#19264=EDGE_CURVE('',#14854,#14854,#1869,.T.);
#19265=EDGE_CURVE('',#14840,#14854,#9686,.T.);
#19266=EDGE_CURVE('',#14836,#14838,#1870,.F.);
#19267=EDGE_CURVE('',#14855,#14855,#1871,.T.);
#19268=EDGE_CURVE('',#14855,#14837,#9687,.T.);
#27941=ORIENTED_EDGE('',*,*,#19192,.F.);
#27942=ORIENTED_EDGE('',*,*,#19193,.T.);
#27943=ORIENTED_EDGE('',*,*,#19194,.T.);
#27944=ORIENTED_EDGE('',*,*,#19195,.T.);
#27945=ORIENTED_EDGE('',*,*,#19196,.F.);
#27946=ORIENTED_EDGE('',*,*,#19197,.T.);
#27947=ORIENTED_EDGE('',*,*,#19192,.T.);
#27948=ORIENTED_EDGE('',*,*,#19198,.T.);
#27949=ORIENTED_EDGE('',*,*,#19199,.F.);
#27950=ORIENTED_EDGE('',*,*,#19200,.T.);
#27951=ORIENTED_EDGE('',*,*,#19196,.T.);
#27952=ORIENTED_EDGE('',*,*,#19201,.T.);
#27953=ORIENTED_EDGE('',*,*,#19202,.F.);
#27954=ORIENTED_EDGE('',*,*,#19203,.T.);
#27955=ORIENTED_EDGE('',*,*,#19199,.T.);
#27956=ORIENTED_EDGE('',*,*,#19204,.T.);
#27957=ORIENTED_EDGE('',*,*,#19205,.F.);
#27958=ORIENTED_EDGE('',*,*,#19206,.T.);
#27959=ORIENTED_EDGE('',*,*,#19202,.T.);
#27960=ORIENTED_EDGE('',*,*,#19207,.T.);
#27961=ORIENTED_EDGE('',*,*,#19208,.F.);
#27962=ORIENTED_EDGE('',*,*,#19209,.T.);
#27963=ORIENTED_EDGE('',*,*,#19205,.T.);
#27964=ORIENTED_EDGE('',*,*,#19210,.T.);
#27965=ORIENTED_EDGE('',*,*,#19211,.F.);
#27966=ORIENTED_EDGE('',*,*,#19212,.T.);
#27967=ORIENTED_EDGE('',*,*,#19208,.T.);
#27968=ORIENTED_EDGE('',*,*,#19213,.T.);
#27969=ORIENTED_EDGE('',*,*,#19214,.F.);
#27970=ORIENTED_EDGE('',*,*,#19215,.T.);
#27971=ORIENTED_EDGE('',*,*,#19216,.F.);
#27972=ORIENTED_EDGE('',*,*,#19217,.F.);
#27973=ORIENTED_EDGE('',*,*,#19218,.F.);
#27974=ORIENTED_EDGE('',*,*,#19219,.T.);
#27975=ORIENTED_EDGE('',*,*,#19214,.T.);
#27976=ORIENTED_EDGE('',*,*,#19220,.F.);
#27977=ORIENTED_EDGE('',*,*,#19221,.F.);
#27978=ORIENTED_EDGE('',*,*,#19222,.T.);
#27979=ORIENTED_EDGE('',*,*,#19218,.T.);
#27980=ORIENTED_EDGE('',*,*,#19223,.F.);
#27981=ORIENTED_EDGE('',*,*,#19224,.F.);
#27982=ORIENTED_EDGE('',*,*,#19225,.T.);
#27983=ORIENTED_EDGE('',*,*,#19221,.T.);
#27984=ORIENTED_EDGE('',*,*,#19226,.F.);
#27985=ORIENTED_EDGE('',*,*,#19227,.F.);
#27986=ORIENTED_EDGE('',*,*,#19228,.T.);
#27987=ORIENTED_EDGE('',*,*,#19224,.T.);
#27988=ORIENTED_EDGE('',*,*,#19229,.F.);
#27989=ORIENTED_EDGE('',*,*,#19230,.F.);
#27990=ORIENTED_EDGE('',*,*,#19231,.T.);
#27991=ORIENTED_EDGE('',*,*,#19227,.T.);
#27992=ORIENTED_EDGE('',*,*,#19232,.F.);
#27993=ORIENTED_EDGE('',*,*,#19216,.T.);
#27994=ORIENTED_EDGE('',*,*,#19233,.T.);
#27995=ORIENTED_EDGE('',*,*,#19234,.F.);
#27996=ORIENTED_EDGE('',*,*,#19235,.F.);
#27997=ORIENTED_EDGE('',*,*,#19236,.T.);
#27998=ORIENTED_EDGE('',*,*,#19236,.F.);
#27999=ORIENTED_EDGE('',*,*,#19237,.F.);
#28000=ORIENTED_EDGE('',*,*,#19213,.F.);
#28001=ORIENTED_EDGE('',*,*,#19210,.F.);
#28002=ORIENTED_EDGE('',*,*,#19207,.F.);
#28003=ORIENTED_EDGE('',*,*,#19204,.F.);
#28004=ORIENTED_EDGE('',*,*,#19201,.F.);
#28005=ORIENTED_EDGE('',*,*,#19198,.F.);
#28006=ORIENTED_EDGE('',*,*,#19195,.F.);
#28007=ORIENTED_EDGE('',*,*,#19238,.F.);
#28008=ORIENTED_EDGE('',*,*,#19239,.T.);
#28009=ORIENTED_EDGE('',*,*,#19232,.T.);
#28010=ORIENTED_EDGE('',*,*,#19229,.T.);
#28011=ORIENTED_EDGE('',*,*,#19226,.T.);
#28012=ORIENTED_EDGE('',*,*,#19223,.T.);
#28013=ORIENTED_EDGE('',*,*,#19220,.T.);
#28014=ORIENTED_EDGE('',*,*,#19217,.T.);
#28015=ORIENTED_EDGE('',*,*,#19240,.T.);
#28016=ORIENTED_EDGE('',*,*,#19241,.T.);
#28017=ORIENTED_EDGE('',*,*,#19242,.T.);
#28018=ORIENTED_EDGE('',*,*,#19243,.T.);
#28019=ORIENTED_EDGE('',*,*,#19238,.T.);
#28020=ORIENTED_EDGE('',*,*,#19230,.T.);
#28021=ORIENTED_EDGE('',*,*,#19239,.F.);
#28022=ORIENTED_EDGE('',*,*,#19243,.F.);
#28023=ORIENTED_EDGE('',*,*,#19244,.T.);
#28024=ORIENTED_EDGE('',*,*,#19233,.F.);
#28025=ORIENTED_EDGE('',*,*,#19215,.F.);
#28026=ORIENTED_EDGE('',*,*,#19219,.F.);
#28027=ORIENTED_EDGE('',*,*,#19222,.F.);
#28028=ORIENTED_EDGE('',*,*,#19225,.F.);
#28029=ORIENTED_EDGE('',*,*,#19228,.F.);
#28030=ORIENTED_EDGE('',*,*,#19231,.F.);
#28031=ORIENTED_EDGE('',*,*,#19244,.F.);
#28032=ORIENTED_EDGE('',*,*,#19242,.F.);
#28033=ORIENTED_EDGE('',*,*,#19193,.F.);
#28034=ORIENTED_EDGE('',*,*,#19197,.F.);
#28035=ORIENTED_EDGE('',*,*,#19200,.F.);
#28036=ORIENTED_EDGE('',*,*,#19203,.F.);
#28037=ORIENTED_EDGE('',*,*,#19206,.F.);
#28038=ORIENTED_EDGE('',*,*,#19209,.F.);
#28039=ORIENTED_EDGE('',*,*,#19212,.F.);
#28040=ORIENTED_EDGE('',*,*,#19245,.F.);
#28041=ORIENTED_EDGE('',*,*,#19246,.F.);
#28042=ORIENTED_EDGE('',*,*,#19247,.T.);
#28043=ORIENTED_EDGE('',*,*,#19248,.T.);
#28044=ORIENTED_EDGE('',*,*,#19249,.F.);
#28045=ORIENTED_EDGE('',*,*,#19250,.F.);
#28046=ORIENTED_EDGE('',*,*,#19251,.T.);
#28047=ORIENTED_EDGE('',*,*,#19252,.T.);
#28048=ORIENTED_EDGE('',*,*,#19247,.F.);
#28049=ORIENTED_EDGE('',*,*,#19253,.F.);
#28050=ORIENTED_EDGE('',*,*,#19254,.T.);
#28051=ORIENTED_EDGE('',*,*,#19255,.T.);
#28052=ORIENTED_EDGE('',*,*,#19251,.F.);
#28053=ORIENTED_EDGE('',*,*,#19256,.F.);
#28054=ORIENTED_EDGE('',*,*,#19257,.T.);
#28055=ORIENTED_EDGE('',*,*,#19258,.T.);
#28056=ORIENTED_EDGE('',*,*,#19254,.F.);
#28057=ORIENTED_EDGE('',*,*,#19259,.F.);
#28058=ORIENTED_EDGE('',*,*,#19260,.T.);
#28059=ORIENTED_EDGE('',*,*,#19261,.T.);
#28060=ORIENTED_EDGE('',*,*,#19257,.F.);
#28061=ORIENTED_EDGE('',*,*,#19262,.F.);
#28062=ORIENTED_EDGE('',*,*,#19249,.T.);
#28063=ORIENTED_EDGE('',*,*,#19263,.T.);
#28064=ORIENTED_EDGE('',*,*,#19260,.F.);
#28065=ORIENTED_EDGE('',*,*,#19263,.F.);
#28066=ORIENTED_EDGE('',*,*,#19248,.F.);
#28067=ORIENTED_EDGE('',*,*,#19252,.F.);
#28068=ORIENTED_EDGE('',*,*,#19255,.F.);
#28069=ORIENTED_EDGE('',*,*,#19258,.F.);
#28070=ORIENTED_EDGE('',*,*,#19261,.F.);
#28071=ORIENTED_EDGE('',*,*,#19264,.F.);
#28072=ORIENTED_EDGE('',*,*,#19240,.F.);
#28073=ORIENTED_EDGE('',*,*,#19194,.F.);
#28074=ORIENTED_EDGE('',*,*,#19241,.F.);
#28075=ORIENTED_EDGE('',*,*,#19265,.T.);
#28076=ORIENTED_EDGE('',*,*,#19264,.T.);
#28077=ORIENTED_EDGE('',*,*,#19265,.F.);
#28078=ORIENTED_EDGE('',*,*,#19211,.T.);
#28079=ORIENTED_EDGE('',*,*,#19237,.T.);
#28080=ORIENTED_EDGE('',*,*,#19266,.F.);
#28081=ORIENTED_EDGE('',*,*,#19245,.T.);
#28082=ORIENTED_EDGE('',*,*,#19267,.F.);
#28083=ORIENTED_EDGE('',*,*,#19268,.T.);
#28084=ORIENTED_EDGE('',*,*,#19234,.T.);
#28085=ORIENTED_EDGE('',*,*,#19266,.T.);
#28086=ORIENTED_EDGE('',*,*,#19235,.T.);
#28087=ORIENTED_EDGE('',*,*,#19268,.F.);
#28088=ORIENTED_EDGE('',*,*,#19267,.T.);
#28089=ORIENTED_EDGE('',*,*,#19246,.T.);
#28090=ORIENTED_EDGE('',*,*,#19262,.T.);
#28091=ORIENTED_EDGE('',*,*,#19259,.T.);
#28092=ORIENTED_EDGE('',*,*,#19256,.T.);
#28093=ORIENTED_EDGE('',*,*,#19253,.T.);
#28094=ORIENTED_EDGE('',*,*,#19250,.T.);
#28894=PLANE('',#33354);
#28895=PLANE('',#33357);
#28896=PLANE('',#33362);
#28897=PLANE('',#33363);
#28898=PLANE('',#33364);
#28899=PLANE('',#33365);
#28900=PLANE('',#33366);
#28901=PLANE('',#33367);
#28902=PLANE('',#33368);
#28903=PLANE('',#33369);
#28904=PLANE('',#33376);
#30631=ADVANCED_FACE('',(#5303),#1021,.T.);
#30632=ADVANCED_FACE('',(#5304),#1022,.T.);
#30633=ADVANCED_FACE('',(#5305),#1023,.T.);
#30634=ADVANCED_FACE('',(#5306),#1024,.T.);
#30635=ADVANCED_FACE('',(#5307),#1025,.T.);
#30636=ADVANCED_FACE('',(#5308),#1026,.T.);
#30637=ADVANCED_FACE('',(#5309),#1027,.T.);
#30638=ADVANCED_FACE('',(#5310),#1028,.T.);
#30639=ADVANCED_FACE('',(#5311),#1029,.T.);
#30640=ADVANCED_FACE('',(#5312),#1030,.T.);
#30641=ADVANCED_FACE('',(#5313),#1031,.T.);
#30642=ADVANCED_FACE('',(#5314),#1032,.T.);
#30643=ADVANCED_FACE('',(#5315),#1033,.T.);
#30644=ADVANCED_FACE('',(#5316),#28894,.F.);
#30645=ADVANCED_FACE('',(#5317),#431,.F.);
#30646=ADVANCED_FACE('',(#5318),#28895,.T.);
#30647=ADVANCED_FACE('',(#5319),#1034,.T.);
#30648=ADVANCED_FACE('',(#5320),#432,.F.);
#30649=ADVANCED_FACE('',(#5321),#28896,.F.);
#30650=ADVANCED_FACE('',(#5322),#28897,.F.);
#30651=ADVANCED_FACE('',(#5323),#28898,.F.);
#30652=ADVANCED_FACE('',(#5324),#28899,.F.);
#30653=ADVANCED_FACE('',(#5325),#28900,.F.);
#30654=ADVANCED_FACE('',(#5326),#28901,.F.);
#30655=ADVANCED_FACE('',(#5327),#28902,.F.);
#30656=ADVANCED_FACE('',(#5328),#28903,.T.);
#30657=ADVANCED_FACE('',(#5329),#2081,.T.);
#30658=ADVANCED_FACE('',(#5330),#1035,.T.);
#30659=ADVANCED_FACE('',(#5331),#2082,.T.);
#30660=ADVANCED_FACE('',(#5332,#3576),#28904,.T.);
#30679=CLOSED_SHELL('',(#30631,#30632,#30633,#30634,#30635,#30636,#30637,
#30638,#30639,#30640,#30641,#30642,#30643,#30644,#30645,#30646,#30647,#30648,
#30649,#30650,#30651,#30652,#30653,#30654,#30655,#30656,#30657,#30658,#30659,
#30660));
#33338=AXIS2_PLACEMENT_3D('',#81021,#40582,#40583);
#33339=AXIS2_PLACEMENT_3D('',#81022,#40584,#40585);
#33340=AXIS2_PLACEMENT_3D('',#81038,#40587,#40588);
#33341=AXIS2_PLACEMENT_3D('',#81046,#40589,#40590);
#33342=AXIS2_PLACEMENT_3D('',#81094,#40592,#40593);
#33343=AXIS2_PLACEMENT_3D('',#81142,#40595,#40596);
#33344=AXIS2_PLACEMENT_3D('',#81196,#40598,#40599);
#33345=AXIS2_PLACEMENT_3D('',#81244,#40601,#40602);
#33346=AXIS2_PLACEMENT_3D('',#81292,#40604,#40605);
#33347=AXIS2_PLACEMENT_3D('',#81340,#40607,#40608);
#33348=AXIS2_PLACEMENT_3D('',#81356,#40610,#40611);
#33349=AXIS2_PLACEMENT_3D('',#81366,#40612,#40613);
#33350=AXIS2_PLACEMENT_3D('',#81390,#40615,#40616);
#33351=AXIS2_PLACEMENT_3D('',#81414,#40618,#40619);
#33352=AXIS2_PLACEMENT_3D('',#81439,#40621,#40622);
#33353=AXIS2_PLACEMENT_3D('',#81464,#40624,#40625);
#33354=AXIS2_PLACEMENT_3D('',#81488,#40627,#40628);
#33355=AXIS2_PLACEMENT_3D('',#81576,#40629,#40630);
#33356=AXIS2_PLACEMENT_3D('',#81578,#40631,#40632);
#33357=AXIS2_PLACEMENT_3D('',#81960,#40633,#40634);
#33358=AXIS2_PLACEMENT_3D('',#81962,#40635,#40636);
#33359=AXIS2_PLACEMENT_3D('',#81963,#40637,#40638);
#33360=AXIS2_PLACEMENT_3D('',#82050,#40639,#40640);
#33361=AXIS2_PLACEMENT_3D('',#82051,#40641,#40642);
#33362=AXIS2_PLACEMENT_3D('',#82258,#40643,#40644);
#33363=AXIS2_PLACEMENT_3D('',#82267,#40649,#40650);
#33364=AXIS2_PLACEMENT_3D('',#82273,#40654,#40655);
#33365=AXIS2_PLACEMENT_3D('',#82279,#40659,#40660);
#33366=AXIS2_PLACEMENT_3D('',#82285,#40664,#40665);
#33367=AXIS2_PLACEMENT_3D('',#82291,#40669,#40670);
#33368=AXIS2_PLACEMENT_3D('',#82294,#40673,#40674);
#33369=AXIS2_PLACEMENT_3D('',#82295,#40675,#40676);
#33370=AXIS2_PLACEMENT_3D('',#82297,#40677,#40678);
#33371=AXIS2_PLACEMENT_3D('',#82298,#40679,#40680);
#33372=AXIS2_PLACEMENT_3D('',#82300,#40682,#40683);
#33373=AXIS2_PLACEMENT_3D('',#82301,#40684,#40685);
#33374=AXIS2_PLACEMENT_3D('',#82302,#40686,#40687);
#33375=AXIS2_PLACEMENT_3D('',#82304,#40688,#40689);
#33376=AXIS2_PLACEMENT_3D('',#82306,#40691,#40692);
#40582=DIRECTION('axis',(0.,0.,1.));
#40583=DIRECTION('refdir',(1.,0.,0.));
#40584=DIRECTION('center_axis',(1.,0.,0.));
#40585=DIRECTION('ref_axis',(0.,1.,0.));
#40586=DIRECTION('',(-1.,0.,0.));
#40587=DIRECTION('center_axis',(1.,0.,0.));
#40588=DIRECTION('ref_axis',(0.,1.,0.));
#40589=DIRECTION('center_axis',(1.,0.,0.));
#40590=DIRECTION('ref_axis',(0.,1.,0.));
#40591=DIRECTION('',(-1.,0.,0.));
#40592=DIRECTION('center_axis',(1.,0.,0.));
#40593=DIRECTION('ref_axis',(0.,1.,0.));
#40594=DIRECTION('',(-1.,0.,0.));
#40595=DIRECTION('center_axis',(1.,0.,0.));
#40596=DIRECTION('ref_axis',(0.,1.,0.));
#40597=DIRECTION('',(-1.,0.,0.));
#40598=DIRECTION('center_axis',(1.,0.,0.));
#40599=DIRECTION('ref_axis',(0.,1.,0.));
#40600=DIRECTION('',(-1.,0.,0.));
#40601=DIRECTION('center_axis',(1.,0.,0.));
#40602=DIRECTION('ref_axis',(0.,1.,0.));
#40603=DIRECTION('',(-1.,0.,0.));
#40604=DIRECTION('center_axis',(1.,0.,0.));
#40605=DIRECTION('ref_axis',(0.,1.,0.));
#40606=DIRECTION('',(-1.,0.,0.));
#40607=DIRECTION('center_axis',(1.,0.,0.));
#40608=DIRECTION('ref_axis',(5.89165264606854E-17,1.,2.23777851519704E-14));
#40609=DIRECTION('',(1.,0.,0.));
#40610=DIRECTION('center_axis',(1.,0.,0.));
#40611=DIRECTION('ref_axis',(5.89165264606854E-17,1.,2.23777851519704E-14));
#40612=DIRECTION('center_axis',(1.,0.,0.));
#40613=DIRECTION('ref_axis',(5.89165264606854E-17,1.,2.23777851519704E-14));
#40614=DIRECTION('',(1.,0.,0.));
#40615=DIRECTION('center_axis',(1.,0.,0.));
#40616=DIRECTION('ref_axis',(5.89165264606854E-17,1.,2.23777851519704E-14));
#40617=DIRECTION('',(1.,0.,0.));
#40618=DIRECTION('center_axis',(1.,0.,0.));
#40619=DIRECTION('ref_axis',(5.89165264606854E-17,1.,2.23777851519704E-14));
#40620=DIRECTION('',(1.,0.,0.));
#40621=DIRECTION('center_axis',(1.,0.,0.));
#40622=DIRECTION('ref_axis',(5.89165264606854E-17,1.,2.23777851519704E-14));
#40623=DIRECTION('',(1.,0.,0.));
#40624=DIRECTION('center_axis',(1.,0.,0.));
#40625=DIRECTION('ref_axis',(5.89165264606854E-17,1.,2.23777851519704E-14));
#40626=DIRECTION('',(1.,0.,0.));
#40627=DIRECTION('center_axis',(1.,0.,0.));
#40628=DIRECTION('ref_axis',(0.,0.,-1.));
#40629=DIRECTION('center_axis',(-1.,0.,0.));
#40630=DIRECTION('ref_axis',(0.,1.,0.));
#40631=DIRECTION('center_axis',(-1.,0.,0.));
#40632=DIRECTION('ref_axis',(0.,1.,0.));
#40633=DIRECTION('center_axis',(1.,0.,0.));
#40634=DIRECTION('ref_axis',(0.,0.,-1.));
#40635=DIRECTION('center_axis',(1.,0.,0.));
#40636=DIRECTION('ref_axis',(0.,1.,0.));
#40637=DIRECTION('center_axis',(1.,0.,0.));
#40638=DIRECTION('ref_axis',(0.,1.,0.));
#40639=DIRECTION('center_axis',(-1.,0.,0.));
#40640=DIRECTION('ref_axis',(5.89165264606854E-17,1.,2.23777851519704E-14));
#40641=DIRECTION('center_axis',(1.,0.,0.));
#40642=DIRECTION('ref_axis',(5.89165264606854E-17,1.,2.23777851519704E-14));
#40643=DIRECTION('center_axis',(0.,0.5,0.866025403784439));
#40644=DIRECTION('ref_axis',(0.,0.866025403784439,-0.5));
#40645=DIRECTION('',(0.,0.866025403784439,-0.5));
#40646=DIRECTION('',(-1.,0.,0.));
#40647=DIRECTION('',(0.,0.866025403784439,-0.5));
#40648=DIRECTION('',(-1.,0.,0.));
#40649=DIRECTION('center_axis',(0.,-0.5,0.866025403784439));
#40650=DIRECTION('ref_axis',(0.,0.866025403784439,0.5));
#40651=DIRECTION('',(0.,0.866025403784439,0.5));
#40652=DIRECTION('',(-1.,0.,0.));
#40653=DIRECTION('',(0.,0.866025403784439,0.5));
#40654=DIRECTION('center_axis',(0.,-1.,-1.60246890531964E-16));
#40655=DIRECTION('ref_axis',(0.,-1.60246890531964E-16,1.));
#40656=DIRECTION('',(0.,-1.60246890531964E-16,1.));
#40657=DIRECTION('',(-1.,0.,0.));
#40658=DIRECTION('',(0.,-1.60246890531964E-16,1.));
#40659=DIRECTION('center_axis',(0.,-0.5,-0.866025403784439));
#40660=DIRECTION('ref_axis',(0.,-0.866025403784439,0.5));
#40661=DIRECTION('',(0.,-0.866025403784439,0.5));
#40662=DIRECTION('',(-1.,0.,0.));
#40663=DIRECTION('',(0.,-0.866025403784439,0.5));
#40664=DIRECTION('center_axis',(0.,0.5,-0.866025403784439));
#40665=DIRECTION('ref_axis',(0.,-0.866025403784439,-0.5));
#40666=DIRECTION('',(0.,-0.866025403784439,-0.5));
#40667=DIRECTION('',(-1.,0.,0.));
#40668=DIRECTION('',(0.,-0.866025403784439,-0.5));
#40669=DIRECTION('center_axis',(0.,1.,-3.20493781063927E-16));
#40670=DIRECTION('ref_axis',(0.,-3.20493781063927E-16,-1.));
#40671=DIRECTION('',(0.,-3.20493781063927E-16,-1.));
#40672=DIRECTION('',(0.,-3.20493781063927E-16,-1.));
#40673=DIRECTION('center_axis',(-1.,0.,0.));
#40674=DIRECTION('ref_axis',(0.,0.,1.));
#40675=DIRECTION('center_axis',(-1.,0.,0.));
#40676=DIRECTION('ref_axis',(0.,0.,1.));
#40677=DIRECTION('center_axis',(1.,0.,0.));
#40678=DIRECTION('ref_axis',(0.,0.,-1.));
#40679=DIRECTION('center_axis',(1.,0.,0.));
#40680=DIRECTION('ref_axis',(0.,1.,0.));
#40681=DIRECTION('',(-0.707106781186548,0.707106781186547,8.65956056235493E-17));
#40682=DIRECTION('center_axis',(1.,0.,0.));
#40683=DIRECTION('ref_axis',(0.,1.,0.));
#40684=DIRECTION('center_axis',(-1.,0.,0.));
#40685=DIRECTION('ref_axis',(0.,1.,0.));
#40686=DIRECTION('center_axis',(-1.,0.,0.));
#40687=DIRECTION('ref_axis',(0.,1.,0.));
#40688=DIRECTION('center_axis',(1.,0.,0.));
#40689=DIRECTION('ref_axis',(0.,0.,-1.));
#40690=DIRECTION('',(-0.707106781186548,-0.707106781186547,-8.65956056235493E-17));
#40691=DIRECTION('center_axis',(1.,0.,0.));
#40692=DIRECTION('ref_axis',(0.,0.,-1.));
#81021=CARTESIAN_POINT('',(0.,0.,0.));
#81022=CARTESIAN_POINT('Origin',(2.075,0.,0.));
#81023=CARTESIAN_POINT('',(0.574155045842906,-1.46519261812194,0.000976835818179873));
#81024=CARTESIAN_POINT('',(0.502844954157094,-1.46475946759348,0.00161057725761545));
#81025=CARTESIAN_POINT('',(2.075,-1.4635,-1.79227059055215E-16));
#81026=CARTESIAN_POINT('',(0.4135,0.634777254283071,1.31995703642142));
#81027=CARTESIAN_POINT('Ctrl Pts',(0.574155045842906,-1.46519261812194,
0.000976835818179873));
#81028=CARTESIAN_POINT('Ctrl Pts',(0.57130704891923,-1.46556281925314,0.0531772786997573));
#81029=CARTESIAN_POINT('Ctrl Pts',(0.568459051995553,-1.46301484057674,
0.105338898321017));
#81030=CARTESIAN_POINT('Ctrl Pts',(0.565611055071877,-1.45742890091883,
0.157170235506765));
#81031=CARTESIAN_POINT('Ctrl Pts',(0.539186980530809,-1.4056018484823,0.638067916952109));
#81032=CARTESIAN_POINT('Ctrl Pts',(0.512762905989741,-1.09225610638139,
1.09053368953482));
#81033=CARTESIAN_POINT('Ctrl Pts',(0.486338831448674,-0.660330380719405,
1.30858720339481));
#81034=CARTESIAN_POINT('Ctrl Pts',(0.462059220965782,-0.263457886270657,
1.50894443341694));
#81035=CARTESIAN_POINT('Ctrl Pts',(0.437779610482891,0.233528707448358,
1.51139328602859));
#81036=CARTESIAN_POINT('Ctrl Pts',(0.4135,0.63554741399093,1.32087379520599));
#81037=CARTESIAN_POINT('',(0.4135,-0.634007094575215,1.31904027763685));
#81038=CARTESIAN_POINT('Origin',(0.4135,0.,0.));
#81039=CARTESIAN_POINT('Ctrl Pts',(0.4135,-0.634007094575211,1.31904027763685));
#81040=CARTESIAN_POINT('Ctrl Pts',(0.439924074541068,-1.07200063648892,
1.10851523328497));
#81041=CARTESIAN_POINT('Ctrl Pts',(0.466348149082135,-1.393162466651,0.66456818150847));
#81042=CARTESIAN_POINT('Ctrl Pts',(0.492772223623203,-1.4539947208087,0.185460774447188));
#81043=CARTESIAN_POINT('Ctrl Pts',(0.496129800467833,-1.46172437535721,
0.124582958895325));
#81044=CARTESIAN_POINT('Ctrl Pts',(0.499487377312464,-1.4652508704938,0.0631374607139664));
#81045=CARTESIAN_POINT('Ctrl Pts',(0.502844954157094,-1.46475946759348,
0.00161057725761545));
#81046=CARTESIAN_POINT('Origin',(2.075,0.,0.));
#81047=CARTESIAN_POINT('',(1.07415504584291,-1.46139381528846,0.000649084939641151));
#81048=CARTESIAN_POINT('',(1.00284495415709,-1.46127859184819,0.000519472235833149));
#81049=CARTESIAN_POINT('',(2.075,-1.4635,-1.79227059055215E-16));
#81050=CARTESIAN_POINT('Ctrl Pts',(1.07415504584291,-1.46139381528846,0.000649084939641151));
#81051=CARTESIAN_POINT('Ctrl Pts',(1.06318482949897,-1.46220383399087,0.203077133365655));
#81052=CARTESIAN_POINT('Ctrl Pts',(1.05221461315503,-1.4230119511318,0.405204867450792));
#81053=CARTESIAN_POINT('Ctrl Pts',(1.0412443968111,-1.34229994073582,0.589109347613649));
#81054=CARTESIAN_POINT('Ctrl Pts',(1.01482032227003,-1.14788807936524,1.03208198734153));
#81055=CARTESIAN_POINT('Ctrl Pts',(0.988396247728961,-0.71258117373777,
1.36932538632444));
#81056=CARTESIAN_POINT('Ctrl Pts',(0.961972173187893,-0.235083460125689,
1.44690837412835));
#81057=CARTESIAN_POINT('Ctrl Pts',(0.935548098646825,0.242414253486394,
1.52449136193227));
#81058=CARTESIAN_POINT('Ctrl Pts',(0.909124024105757,0.762102775083091,
1.34241393855718));
#81059=CARTESIAN_POINT('Ctrl Pts',(0.882699949564689,1.08675402559799,0.983767539938644));
#81060=CARTESIAN_POINT('Ctrl Pts',(0.856275875023622,1.4114052761129,0.625121141320107));
#81061=CARTESIAN_POINT('Ctrl Pts',(0.829851800482554,1.54101925554601,0.0899057674581173));
#81062=CARTESIAN_POINT('Ctrl Pts',(0.803427725941486,1.41643784418256,-0.377524557756998));
#81063=CARTESIAN_POINT('Ctrl Pts',(0.777003651400418,1.29185643281911,-0.844954882972116));
#81064=CARTESIAN_POINT('Ctrl Pts',(0.750579576859351,0.913079630659097,
-1.24460015954036));
#81065=CARTESIAN_POINT('Ctrl Pts',(0.724155502318283,0.452995311679302,
-1.39411299623214));
#81066=CARTESIAN_POINT('Ctrl Pts',(0.697731427777215,-0.00708900730049256,
-1.54362583292391));
#81067=CARTESIAN_POINT('Ctrl Pts',(0.671307353236147,-0.548480843100068,
-1.44300622973923));
#81068=CARTESIAN_POINT('Ctrl Pts',(0.64488327869508,-0.924022579613784,
-1.13803163299289));
#81069=CARTESIAN_POINT('Ctrl Pts',(0.621307201077688,-1.25908828323405,
-0.865927315657216));
#81070=CARTESIAN_POINT('Ctrl Pts',(0.597731123460297,-1.46212804648194,
-0.431145011929348));
#81071=CARTESIAN_POINT('Ctrl Pts',(0.574155045842906,-1.46519261812194,
0.000976835818179873));
#81072=CARTESIAN_POINT('Ctrl Pts',(0.502844954157094,-1.46475946759348,
0.00161057725761545));
#81073=CARTESIAN_POINT('Ctrl Pts',(0.525911451853531,-1.46138353775099,
-0.421078100079624));
#81074=CARTESIAN_POINT('Ctrl Pts',(0.548977949549969,-1.2683761840885,-0.847607891709197));
#81075=CARTESIAN_POINT('Ctrl Pts',(0.572044447246407,-0.945806624145029,
-1.12030156148761));
#81076=CARTESIAN_POINT('Ctrl Pts',(0.598468521787474,-0.576283595170322,
-1.43268872801506));
#81077=CARTESIAN_POINT('Ctrl Pts',(0.624892596328542,-0.0367348590675789,
-1.5431952987239));
#81078=CARTESIAN_POINT('Ctrl Pts',(0.651316670869609,0.426181990272789,
-1.40242879098034));
#81079=CARTESIAN_POINT('Ctrl Pts',(0.677740745410677,0.889098839613157,
-1.26166228323678));
#81080=CARTESIAN_POINT('Ctrl Pts',(0.704164819951745,1.27538380219115,-0.869622697040829));
#81081=CARTESIAN_POINT('Ctrl Pts',(0.730588894492813,1.40889782546728,-0.404732685395172));
#81082=CARTESIAN_POINT('Ctrl Pts',(0.757012969033881,1.54241184874341,0.0601573262504863));
#81083=CARTESIAN_POINT('Ctrl Pts',(0.783437043574948,1.42315493271767,0.597897763345852));
#81084=CARTESIAN_POINT('Ctrl Pts',(0.809861118116016,1.1054653199822,0.962746225793369));
#81085=CARTESIAN_POINT('Ctrl Pts',(0.836285192657083,0.787775707246719,
1.32759468824088));
#81086=CARTESIAN_POINT('Ctrl Pts',(0.862709267198151,0.271653397801502,
1.51955117604055));
#81087=CARTESIAN_POINT('Ctrl Pts',(0.889133341739219,-0.207253044667741,
1.45113831243121));
#81088=CARTESIAN_POINT('Ctrl Pts',(0.915557416280287,-0.686159487136987,
1.38272544882186));
#81089=CARTESIAN_POINT('Ctrl Pts',(0.941981490821354,-1.12785006263026,
1.0539432338035));
#81090=CARTESIAN_POINT('Ctrl Pts',(0.968405565362422,-1.33073196102483,
0.614795628754564));
#81091=CARTESIAN_POINT('Ctrl Pts',(0.979885361627313,-1.41887290445823,
0.4240103269518));
#81092=CARTESIAN_POINT('Ctrl Pts',(0.991365157892203,-1.46194059597963,
0.212394429344695));
#81093=CARTESIAN_POINT('Ctrl Pts',(1.00284495415709,-1.46127859184819,0.000519472235833149));
#81094=CARTESIAN_POINT('Origin',(2.075,0.,0.));
#81095=CARTESIAN_POINT('',(1.57415504584291,-1.46286099658906,-0.00129511982714603));
#81096=CARTESIAN_POINT('',(1.50284495415709,-1.46313245043143,-0.00132110950983211));
#81097=CARTESIAN_POINT('',(2.075,-1.4635,-1.79227059055215E-16));
#81098=CARTESIAN_POINT('Ctrl Pts',(1.57415504584291,-1.46286099658906,-0.00129511982714603));
#81099=CARTESIAN_POINT('Ctrl Pts',(1.55506261007871,-1.45984286410086,0.350117793684843));
#81100=CARTESIAN_POINT('Ctrl Pts',(1.53597017431451,-1.33270149288247,0.703490485179472));
#81101=CARTESIAN_POINT('Ctrl Pts',(1.51687773855032,-1.10228477898897,0.966326030701892));
#81102=CARTESIAN_POINT('Ctrl Pts',(1.49045366400925,-0.783386315816066,
1.3300924004152));
#81103=CARTESIAN_POINT('Ctrl Pts',(1.46402958946818,-0.266666330116682,
1.52043696781344));
#81104=CARTESIAN_POINT('Ctrl Pts',(1.43760551492711,0.212006026409088,1.45047264850784));
#81105=CARTESIAN_POINT('Ctrl Pts',(1.41118144038604,0.690678382934858,1.38050832920223));
#81106=CARTESIAN_POINT('Ctrl Pts',(1.38475736584498,1.13130311028701,1.05023512319278));
#81107=CARTESIAN_POINT('Ctrl Pts',(1.35833329130391,1.33274643432974,0.610413666753209));
#81108=CARTESIAN_POINT('Ctrl Pts',(1.33190921676284,1.53418975837247,0.170592210313635));
#81109=CARTESIAN_POINT('Ctrl Pts',(1.30548514222177,1.49645167910578,-0.378777496556064));
#81110=CARTESIAN_POINT('Ctrl Pts',(1.2790610676807,1.23675879853513,-0.786921626060999));
#81111=CARTESIAN_POINT('Ctrl Pts',(1.25263699313964,0.977065917964476,-1.19506575556593));
#81112=CARTESIAN_POINT('Ctrl Pts',(1.22621291859857,0.495418236089865,-1.46198430770611));
#81113=CARTESIAN_POINT('Ctrl Pts',(1.1997888440575,0.0116750633943819,-1.46583761597847));
#81114=CARTESIAN_POINT('Ctrl Pts',(1.17336476951643,-0.472068109301102,
-1.46969092425084));
#81115=CARTESIAN_POINT('Ctrl Pts',(1.14694069497537,-0.957906772817458,
-1.2104789886554));
#81116=CARTESIAN_POINT('Ctrl Pts',(1.1205166204343,-1.22406769601878,-0.806522080621249));
#81117=CARTESIAN_POINT('Ctrl Pts',(1.10506276223717,-1.37972927494667,-0.570271885186438));
#81118=CARTESIAN_POINT('Ctrl Pts',(1.08960890404004,-1.46025273349283,-0.284513418462271));
#81119=CARTESIAN_POINT('Ctrl Pts',(1.07415504584291,-1.46139381528846,0.000649084939641151));
#81120=CARTESIAN_POINT('Ctrl Pts',(1.00284495415709,-1.46127859184819,0.000519472235833149));
#81121=CARTESIAN_POINT('Ctrl Pts',(1.01778923243327,-1.46041680181882,-0.275297122913305));
#81122=CARTESIAN_POINT('Ctrl Pts',(1.03273351070945,-1.38544822458409,-0.551552734778286));
#81123=CARTESIAN_POINT('Ctrl Pts',(1.04767778898562,-1.23933685982455,-0.782864800020116));
#81124=CARTESIAN_POINT('Ctrl Pts',(1.07410186352669,-0.980986638933794,
-1.19186462866637));
#81125=CARTESIAN_POINT('Ctrl Pts',(1.10052593806776,-0.500212975856397,
-1.4603512908794));
#81126=CARTESIAN_POINT('Ctrl Pts',(1.12695001260883,-0.0164840723619047,
-1.46578875316014));
#81127=CARTESIAN_POINT('Ctrl Pts',(1.1533740871499,0.467244831132591,-1.47122621544088));
#81128=CARTESIAN_POINT('Ctrl Pts',(1.17979816169096,0.953928975044182,-1.21361447778934));
#81129=CARTESIAN_POINT('Ctrl Pts',(1.20622223623203,1.2214137186877,-0.810535480622874));
#81130=CARTESIAN_POINT('Ctrl Pts',(1.2326463107731,1.48889846233122,-0.407456483456409));
#81131=CARTESIAN_POINT('Ctrl Pts',(1.25907038531417,1.53718380570666,0.141089773224978));
#81132=CARTESIAN_POINT('Ctrl Pts',(1.28549445985523,1.34422666083829,0.584700402760684));
#81133=CARTESIAN_POINT('Ctrl Pts',(1.3119185343963,1.15126951596991,1.02831103229639));
#81134=CARTESIAN_POINT('Ctrl Pts',(1.33834260893737,0.717069882857724,1.36698603468642));
#81135=CARTESIAN_POINT('Ctrl Pts',(1.36476668347844,0.239829664321294,1.44613216920364));
#81136=CARTESIAN_POINT('Ctrl Pts',(1.3911907580195,-0.237410554215136,1.52527830372087));
#81137=CARTESIAN_POINT('Ctrl Pts',(1.41761483256057,-0.757691358175806,
1.3448955703653));
#81138=CARTESIAN_POINT('Ctrl Pts',(1.44403890710164,-1.08351870931689,0.987322372169865));
#81139=CARTESIAN_POINT('Ctrl Pts',(1.46364092278679,-1.32522529539969,0.722065951222254));
#81140=CARTESIAN_POINT('Ctrl Pts',(1.48324293847194,-1.45992355989755,0.359301083042489));
#81141=CARTESIAN_POINT('Ctrl Pts',(1.50284495415709,-1.46313245043143,-0.00132110950983211));
#81142=CARTESIAN_POINT('Origin',(2.075,0.,0.));
#81143=CARTESIAN_POINT('',(2.07415504584291,-1.46582439386645,0.000266631823466895));
#81144=CARTESIAN_POINT('',(2.00284495415709,-1.46572742945109,0.000432510777846343));
#81145=CARTESIAN_POINT('',(2.075,-1.4635,-1.79227059055215E-16));
#81146=CARTESIAN_POINT('Ctrl Pts',(2.07415504584291,-1.46582439386645,0.000266631823466895));
#81147=CARTESIAN_POINT('Ctrl Pts',(2.07336446519952,-1.4658608176029,0.0147417778359328));
#81148=CARTESIAN_POINT('Ctrl Pts',(2.07257388455613,-1.46566489447349,0.0292159135494899));
#81149=CARTESIAN_POINT('Ctrl Pts',(2.07178330391274,-1.46523358600562,0.0436830317182805));
#81150=CARTESIAN_POINT('Ctrl Pts',(2.04535922937167,-1.45081769156067,0.527226629810276));
#81151=CARTESIAN_POINT('Ctrl Pts',(2.0189351548306,-1.17344365284929,1.00293065488095));
#81152=CARTESIAN_POINT('Ctrl Pts',(1.99251108028953,-0.759725478262044,
1.25364862470184));
#81153=CARTESIAN_POINT('Ctrl Pts',(1.96608700574846,-0.346007303674802,
1.50436659452273));
#81154=CARTESIAN_POINT('Ctrl Pts',(1.9396629312074,0.2040550067883,1.53009850909383));
#81155=CARTESIAN_POINT('Ctrl Pts',(1.91323885666633,0.639372355957431,1.31909842667499));
#81156=CARTESIAN_POINT('Ctrl Pts',(1.88681478212526,1.07468970512656,1.10809834425614));
#81157=CARTESIAN_POINT('Ctrl Pts',(1.86039070758419,1.39526209300172,0.660366264847353));
#81158=CARTESIAN_POINT('Ctrl Pts',(1.83396663304313,1.45475658686102,0.180280192601334));
#81159=CARTESIAN_POINT('Ctrl Pts',(1.80754255850206,1.51425108072031,-0.299805879644685));
#81160=CARTESIAN_POINT('Ctrl Pts',(1.78111848396099,1.31266768056373,-0.812245944727934));
#81161=CARTESIAN_POINT('Ctrl Pts',(1.75469440941992,0.942023952429685,-1.12312446186072));
#81162=CARTESIAN_POINT('Ctrl Pts',(1.72827033487886,0.571380224295636,-1.4340029789935));
#81163=CARTESIAN_POINT('Ctrl Pts',(1.70184626033779,0.0316761681841161,
-1.54331994817583));
#81164=CARTESIAN_POINT('Ctrl Pts',(1.67542218579672,-0.430727399126193,
-1.40117506038533));
#81165=CARTESIAN_POINT('Ctrl Pts',(1.64899811125565,-0.893130966436502,
-1.25903017259483));
#81166=CARTESIAN_POINT('Ctrl Pts',(1.62257403671458,-1.2782340449456,-0.865423427831514));
#81167=CARTESIAN_POINT('Ctrl Pts',(1.59614996217352,-1.41024711387694,-0.400025969435661));
#81168=CARTESIAN_POINT('Ctrl Pts',(1.58881832339665,-1.44687553519503,-0.270896525476177));
#81169=CARTESIAN_POINT('Ctrl Pts',(1.58148668461978,-1.46401998214006,-0.136240318816841));
#81170=CARTESIAN_POINT('Ctrl Pts',(1.57415504584291,-1.46286099658906,-0.00129511982714603));
#81171=CARTESIAN_POINT('Ctrl Pts',(1.50284495415709,-1.46313245043143,-0.00132110950983211));
#81172=CARTESIAN_POINT('Ctrl Pts',(1.50966701301301,-1.46424923558434,-0.126827887070737));
#81173=CARTESIAN_POINT('Ctrl Pts',(1.51648907186893,-1.4494395291456,-0.252075135634468));
#81174=CARTESIAN_POINT('Ctrl Pts',(1.52331113072484,-1.41767134400802,-0.372862109562419));
#81175=CARTESIAN_POINT('Ctrl Pts',(1.54973520526591,-1.29462272923655,-0.840709730063979));
#81176=CARTESIAN_POINT('Ctrl Pts',(1.57615927980698,-0.917151601372094,
-1.24164130803181));
#81177=CARTESIAN_POINT('Ctrl Pts',(1.60258335434805,-0.457563842382232,
-1.39264248123405));
#81178=CARTESIAN_POINT('Ctrl Pts',(1.62900742888911,0.00202391660763093,
-1.5436436544363));
#81179=CARTESIAN_POINT('Ctrl Pts',(1.65543150343018,0.5437283067229,-1.44471442287297));
#81180=CARTESIAN_POINT('Ctrl Pts',(1.68185557797125,0.920275488657587,-1.14101316666404));
#81181=CARTESIAN_POINT('Ctrl Pts',(1.70827965251232,1.29682267059227,-0.837311910455112));
#81182=CARTESIAN_POINT('Ctrl Pts',(1.73470372705338,1.50821264434637,-0.328838629600589));
#81183=CARTESIAN_POINT('Ctrl Pts',(1.76112780159445,1.45795135754826,0.152301764924768));
#81184=CARTESIAN_POINT('Ctrl Pts',(1.78755187613552,1.40769007075015,0.633442159450128));
#81185=CARTESIAN_POINT('Ctrl Pts',(1.81397595067659,1.09577752339981,1.08724966764632));
#81186=CARTESIAN_POINT('Ctrl Pts',(1.84040002521766,0.664593679489687,1.30657306483852));
#81187=CARTESIAN_POINT('Ctrl Pts',(1.86682409975872,0.233409835579564,1.52589646203071));
#81188=CARTESIAN_POINT('Ctrl Pts',(1.89324817429979,-0.31704530489035,1.51073574821891));
#81189=CARTESIAN_POINT('Ctrl Pts',(1.91967224884086,-0.73550334159657,1.26801135974902));
#81190=CARTESIAN_POINT('Ctrl Pts',(1.94609632338193,-1.15396137830279,1.02528697127912));
#81191=CARTESIAN_POINT('Ctrl Pts',(1.972520397923,-1.44042231124532,0.554998908151132));
#81192=CARTESIAN_POINT('Ctrl Pts',(1.99894447246406,-1.4641241916468,0.0718214210643886));
#81193=CARTESIAN_POINT('Ctrl Pts',(2.00024463302841,-1.46529041035962,0.0480473315191685));
#81194=CARTESIAN_POINT('Ctrl Pts',(2.00154479359275,-1.46582048996688,0.0242420367060462));
#81195=CARTESIAN_POINT('Ctrl Pts',(2.00284495415709,-1.46572742945109,0.000432510777846343));
#81196=CARTESIAN_POINT('Origin',(2.075,0.,0.));
#81197=CARTESIAN_POINT('',(2.57415504584291,-1.4621001751952,0.00110317554495899));
#81198=CARTESIAN_POINT('',(2.50284495415709,-1.46189080583895,0.00100911082079524));
#81199=CARTESIAN_POINT('',(2.075,-1.4635,-1.79227059055215E-16));
#81200=CARTESIAN_POINT('Ctrl Pts',(2.57415504584291,-1.4621001751952,0.00110317554495899));
#81201=CARTESIAN_POINT('Ctrl Pts',(2.56524224577926,-1.46325600427614,0.165366982867302));
#81202=CARTESIAN_POINT('Ctrl Pts',(2.55632944571561,-1.43771198705001,0.329281846754665));
#81203=CARTESIAN_POINT('Ctrl Pts',(2.54741664565196,-1.38391158804006,0.48332822780337));
#81204=CARTESIAN_POINT('Ctrl Pts',(2.52099257111089,-1.22440775718717,0.940034653005688));
#81205=CARTESIAN_POINT('Ctrl Pts',(2.49456849656982,-0.816540414072506,
1.31000063573895));
#81206=CARTESIAN_POINT('Ctrl Pts',(2.46814442202875,-0.34649012402834,1.42434628007155));
#81207=CARTESIAN_POINT('Ctrl Pts',(2.44172034748768,0.123560166015825,1.53869192440415));
#81208=CARTESIAN_POINT('Ctrl Pts',(2.41529627294662,0.655793402989496,1.39741723033608));
#81209=CARTESIAN_POINT('Ctrl Pts',(2.38887219840555,1.00725887392402,1.06501045033488));
#81210=CARTESIAN_POINT('Ctrl Pts',(2.36244812386448,1.35872434485854,0.732603670333682));
#81211=CARTESIAN_POINT('Ctrl Pts',(2.33602404932341,1.5294220497539,0.209064804399345));
#81212=CARTESIAN_POINT('Ctrl Pts',(2.30959997478235,1.44143300464197,-0.266624333721933));
#81213=CARTESIAN_POINT('Ctrl Pts',(2.28317590024128,1.35344395953004,-0.742313471843213));
#81214=CARTESIAN_POINT('Ctrl Pts',(2.25675182570021,1.0067681644108,-1.17015288215143));
#81215=CARTESIAN_POINT('Ctrl Pts',(2.23032775115914,0.559654041834648,-1.35484502332898));
#81216=CARTESIAN_POINT('Ctrl Pts',(2.20390367661807,0.112539919258502,-1.53953716450654));
#81217=CARTESIAN_POINT('Ctrl Pts',(2.17747960207701,-0.435012530774549,
-1.48108203655343));
#81218=CARTESIAN_POINT('Ctrl Pts',(2.15105552753594,-0.833059880701816,
-1.20616288702022));
#81219=CARTESIAN_POINT('Ctrl Pts',(2.12542203363826,-1.21919807068798,-0.939469030591619));
#81220=CARTESIAN_POINT('Ctrl Pts',(2.09978853974058,-1.46464340412969,-0.469070139929011));
#81221=CARTESIAN_POINT('Ctrl Pts',(2.07415504584291,-1.46582439386645,0.000266631823466895));
#81222=CARTESIAN_POINT('Ctrl Pts',(2.00284495415709,-1.46572742945109,0.000432510777846343));
#81223=CARTESIAN_POINT('Ctrl Pts',(2.02796886813382,-1.46392915587056,-0.459655648832342));
#81224=CARTESIAN_POINT('Ctrl Pts',(2.05309278211054,-1.22944698309651,-0.921323729743966));
#81225=CARTESIAN_POINT('Ctrl Pts',(2.07821669608726,-0.856076040177704,
-1.18993771791139));
#81226=CARTESIAN_POINT('Ctrl Pts',(2.10464077062833,-0.46338318044671,-1.47245245875494));
#81227=CARTESIAN_POINT('Ctrl Pts',(2.1310648451694,0.082945366875701,-1.54141502939652));
#81228=CARTESIAN_POINT('Ctrl Pts',(2.15748891971047,0.533524871153222,-1.36534580916677));
#81229=CARTESIAN_POINT('Ctrl Pts',(2.18391299425154,0.984104375430741,-1.18927658893702));
#81230=CARTESIAN_POINT('Ctrl Pts',(2.2103370687926,1.33893483666337,-0.768175577835949));
#81231=CARTESIAN_POINT('Ctrl Pts',(2.23676114333367,1.43604540933339,-0.294264407305756));
#81232=CARTESIAN_POINT('Ctrl Pts',(2.26318521787474,1.53315598200341,0.179646763224435));
#81233=CARTESIAN_POINT('Ctrl Pts',(2.28960929241581,1.37254666611082,0.706368093183742));
#81234=CARTESIAN_POINT('Ctrl Pts',(2.31603336695688,1.02753141629579,1.04546504179445));
#81235=CARTESIAN_POINT('Ctrl Pts',(2.34245744149794,0.682516166480747,1.38456199040515));
#81236=CARTESIAN_POINT('Ctrl Pts',(2.36888151603901,0.153094982743255,1.53603455766725));
#81237=CARTESIAN_POINT('Ctrl Pts',(2.39530559058008,-0.319065158892983,
1.43073945857828));
#81238=CARTESIAN_POINT('Ctrl Pts',(2.42172966512114,-0.791225300529222,
1.32544435948931));
#81239=CARTESIAN_POINT('Ctrl Pts',(2.44815373966221,-1.20612440006421,0.963381594049256));
#81240=CARTESIAN_POINT('Ctrl Pts',(2.47457781420328,-1.37437187360323,0.509823386701214));
#81241=CARTESIAN_POINT('Ctrl Pts',(2.48400019418789,-1.43436608928222,0.348092168144163));
#81242=CARTESIAN_POINT('Ctrl Pts',(2.49342257417249,-1.4629981685089,0.174727162368823));
#81243=CARTESIAN_POINT('Ctrl Pts',(2.50284495415709,-1.46189080583895,0.00100911082079524));
#81244=CARTESIAN_POINT('Origin',(2.075,0.,0.));
#81245=CARTESIAN_POINT('',(3.07415504584291,-1.46191041475934,-0.00101355436836398));
#81246=CARTESIAN_POINT('',(3.00284495415709,-1.46211555199137,-0.00110832896150793));
#81247=CARTESIAN_POINT('',(2.075,-1.4635,-1.79227059055215E-16));
#81248=CARTESIAN_POINT('Ctrl Pts',(3.07415504584291,-1.46191041475934,-0.00101355436836398));
#81249=CARTESIAN_POINT('Ctrl Pts',(3.057120026359,-1.45989180311158,0.313048991404907));
#81250=CARTESIAN_POINT('Ctrl Pts',(3.04008500687508,-1.36064269050357,0.628272692059618));
#81251=CARTESIAN_POINT('Ctrl Pts',(3.02304998739117,-1.17384327638965,0.878009133678142));
#81252=CARTESIAN_POINT('Ctrl Pts',(2.99662591285011,-0.884087127449746,
1.26539080677699));
#81253=CARTESIAN_POINT('Ctrl Pts',(2.97020183830904,-0.383675892838044,
1.49520335760678));
#81254=CARTESIAN_POINT('Ctrl Pts',(2.94377776376797,0.0989770050351939,
1.46253974538111));
#81255=CARTESIAN_POINT('Ctrl Pts',(2.9173536892269,0.581629902908439,1.42987613315544));
#81256=CARTESIAN_POINT('Ctrl Pts',(2.89092961468584,1.04652446404322,1.1347363578743));
#81257=CARTESIAN_POINT('Ctrl Pts',(2.86450554014477,1.28144253601592,0.71184592283405));
#81258=CARTESIAN_POINT('Ctrl Pts',(2.8380814656037,1.51636060798861,0.288955487793809));
#81259=CARTESIAN_POINT('Ctrl Pts',(2.81165739106263,1.52130219079924,-0.261685607005537));
#81260=CARTESIAN_POINT('Ctrl Pts',(2.78523331652156,1.29401468788972,-0.688725062015598));
#81261=CARTESIAN_POINT('Ctrl Pts',(2.7588092419805,1.0667271849802,-1.11576451702566));
#81262=CARTESIAN_POINT('Ctrl Pts',(2.73238516743943,0.607210596350554,-1.41920233224644));
#81263=CARTESIAN_POINT('Ctrl Pts',(2.70596109289836,0.125220624736377,-1.46052653740258));
#81264=CARTESIAN_POINT('Ctrl Pts',(2.6795370183573,-0.356769346877805,-1.50185074255872));
#81265=CARTESIAN_POINT('Ctrl Pts',(2.65311294381622,-0.861232701476513,
-1.28106133765021));
#81266=CARTESIAN_POINT('Ctrl Pts',(2.62668886927516,-1.1578942194803,-0.89894320136026));
#81267=CARTESIAN_POINT('Ctrl Pts',(2.60917759479774,-1.35449225967194,-0.645712929966165));
#81268=CARTESIAN_POINT('Ctrl Pts',(2.59166632032032,-1.45982927938907,-0.321631385556492));
#81269=CARTESIAN_POINT('Ctrl Pts',(2.57415504584291,-1.4621001751952,0.00110317554495899));
#81270=CARTESIAN_POINT('Ctrl Pts',(2.50284495415709,-1.46189080583895,0.00100911082079524));
#81271=CARTESIAN_POINT('Ctrl Pts',(2.51984664871356,-1.45989268626529,-0.312446858497935));
#81272=CARTESIAN_POINT('Ctrl Pts',(2.53684834327002,-1.36106767188624,-0.627052288724924));
#81273=CARTESIAN_POINT('Ctrl Pts',(2.55385003782648,-1.17494880597854,-0.876534820703437));
#81274=CARTESIAN_POINT('Ctrl Pts',(2.58027411236755,-0.88568241727176,-1.264281171504));
#81275=CARTESIAN_POINT('Ctrl Pts',(2.60669818690862,-0.385553792315123,
-1.4947202238491));
#81276=CARTESIAN_POINT('Ctrl Pts',(2.63312226144969,0.0971412829342949,
-1.46266250128816));
#81277=CARTESIAN_POINT('Ctrl Pts',(2.65954633599075,0.579836358183716,-1.43060477872723));
#81278=CARTESIAN_POINT('Ctrl Pts',(2.68597041053182,1.04509788372592,-1.13605028126026));
#81279=CARTESIAN_POINT('Ctrl Pts',(2.71239448507289,1.28054632987947,-0.713455567940678));
#81280=CARTESIAN_POINT('Ctrl Pts',(2.73881855961396,1.51599477603302,-0.290860854621103));
#81281=CARTESIAN_POINT('Ctrl Pts',(2.76524263415503,1.52163014279793,0.25977407455108));
#81282=CARTESIAN_POINT('Ctrl Pts',(2.79166670869609,1.29487961420695,0.687098957268968));
#81283=CARTESIAN_POINT('Ctrl Pts',(2.81809078323716,1.06812908561596,1.11442383998686));
#81284=CARTESIAN_POINT('Ctrl Pts',(2.84451485777823,0.60899266166908,1.41843867625045));
#81285=CARTESIAN_POINT('Ctrl Pts',(2.8709389323193,0.127054938312572,1.46036820791103));
#81286=CARTESIAN_POINT('Ctrl Pts',(2.89736300686036,-0.354882785043935,
1.50229773957161));
#81287=CARTESIAN_POINT('Ctrl Pts',(2.92378708140143,-0.859621807810064,
1.28214196662917));
#81288=CARTESIAN_POINT('Ctrl Pts',(2.9502111559425,-1.15676344772793,0.900397048359602));
#81289=CARTESIAN_POINT('Ctrl Pts',(2.96775575534737,-1.35405440793777,0.646932668539104));
#81290=CARTESIAN_POINT('Ctrl Pts',(2.98530035475223,-1.45982680029096,0.322232288733347));
#81291=CARTESIAN_POINT('Ctrl Pts',(3.00284495415709,-1.46211555199137,-0.00110832896150793));
#81292=CARTESIAN_POINT('Origin',(2.075,0.,0.));
#81293=CARTESIAN_POINT('',(3.57415504584291,-1.46604124392818,-0.000321941105464977));
#81294=CARTESIAN_POINT('',(3.50284495415709,-1.4658722466537,-0.00023313482661453));
#81295=CARTESIAN_POINT('',(2.075,-1.4635,-1.79227059055215E-16));
#81296=CARTESIAN_POINT('Ctrl Pts',(3.57415504584291,-1.46605134156425,-0.000323220338867419));
#81297=CARTESIAN_POINT('Ctrl Pts',(3.54899780693873,-1.46449204195007,0.460439060568385));
#81298=CARTESIAN_POINT('Ctrl Pts',(3.52384056803456,-1.22876388509762,0.922506535519241));
#81299=CARTESIAN_POINT('Ctrl Pts',(3.49868332913039,-0.854425848690436,
1.19096311852186));
#81300=CARTESIAN_POINT('Ctrl Pts',(3.47225925458933,-0.461237382529298,
1.47293829025366));
#81301=CARTESIAN_POINT('Ctrl Pts',(3.44583518004826,0.0848723231897744,
1.54131239917703));
#81302=CARTESIAN_POINT('Ctrl Pts',(3.41941110550719,0.535157675223674,1.36470060702409));
#81303=CARTESIAN_POINT('Ctrl Pts',(3.39298703096612,0.985443027257573,1.18808881487115));
#81304=CARTESIAN_POINT('Ctrl Pts',(3.36656295642505,1.3399040256063,0.766491121641905));
#81305=CARTESIAN_POINT('Ctrl Pts',(3.34013888188399,1.43645708514186,0.292446179449027));
#81306=CARTESIAN_POINT('Ctrl Pts',(3.31371480734292,1.53301014467742,-0.181598762743851));
#81307=CARTESIAN_POINT('Ctrl Pts',(3.28729073280185,1.37165526539981,-0.708090953900364));
#81308=CARTESIAN_POINT('Ctrl Pts',(3.26086665826079,1.026194375012,-1.04674777447125));
#81309=CARTESIAN_POINT('Ctrl Pts',(3.23444258371972,0.68073348462418,-1.38540459504213));
#81310=CARTESIAN_POINT('Ctrl Pts',(3.20801850917865,0.151166583126158,-1.53622604502739));
#81311=CARTESIAN_POINT('Ctrl Pts',(3.18159443463758,-0.320850406538498,
-1.43034120921067));
#81312=CARTESIAN_POINT('Ctrl Pts',(3.15517036009651,-0.792867396203154,
-1.32445637339395));
#81313=CARTESIAN_POINT('Ctrl Pts',(3.12874628555544,-1.20733447403444,-0.961865251775244));
#81314=CARTESIAN_POINT('Ctrl Pts',(3.10232221101438,-1.37501748131604,-0.508094293281935));
#81315=CARTESIAN_POINT('Ctrl Pts',(3.09293315595722,-1.43459894310271,-0.346859488028452));
#81316=CARTESIAN_POINT('Ctrl Pts',(3.08354410090006,-1.46302299675068,-0.174112888739021));
#81317=CARTESIAN_POINT('Ctrl Pts',(3.07415504584291,-1.46191041475934,-0.00101355436836398));
#81318=CARTESIAN_POINT('Ctrl Pts',(3.00284495415709,-1.46211555199137,-0.00110832896150793));
#81319=CARTESIAN_POINT('Ctrl Pts',(3.0117244292933,-1.46327390923554,-0.164753842266872));
#81320=CARTESIAN_POINT('Ctrl Pts',(3.0206039044295,-1.43792533976859,-0.328051057866522));
#81321=CARTESIAN_POINT('Ctrl Pts',(3.0294833795657,-1.38451871835904,-0.481588823801387));
#81322=CARTESIAN_POINT('Ctrl Pts',(3.05590745410677,-1.22558809200266,-0.938495714096107));
#81323=CARTESIAN_POINT('Ctrl Pts',(3.08233152864784,-0.818182582220306,
-1.30897543108885));
#81324=CARTESIAN_POINT('Ctrl Pts',(3.10875560318891,-0.34827766430965,-1.42391077883767));
#81325=CARTESIAN_POINT('Ctrl Pts',(3.13517967772997,0.121627253601006,-1.53884612658648));
#81326=CARTESIAN_POINT('Ctrl Pts',(3.16160375227104,0.65403157963996,-1.39823710509136));
#81327=CARTESIAN_POINT('Ctrl Pts',(3.18802782681211,1.00591707366984,-1.06627352702385));
#81328=CARTESIAN_POINT('Ctrl Pts',(3.21445190135318,1.35780256769973,-0.73430994895634));
#81329=CARTESIAN_POINT('Ctrl Pts',(3.24087597589425,1.52916922972054,-0.210991814316436));
#81330=CARTESIAN_POINT('Ctrl Pts',(3.26730005043531,1.44177276521797,0.264810197511405));
#81331=CARTESIAN_POINT('Ctrl Pts',(3.29372412497638,1.3543763007154,0.740612209339246));
#81332=CARTESIAN_POINT('Ctrl Pts',(3.32014819951745,1.00821670968944,1.16889809835502));
#81333=CARTESIAN_POINT('Ctrl Pts',(3.34657227405851,0.561344663652188,1.35414673718099));
#81334=CARTESIAN_POINT('Ctrl Pts',(3.37299634859958,0.114472617614934,1.53939537600697));
#81335=CARTESIAN_POINT('Ctrl Pts',(3.39942042314065,-0.43311188343362,1.48160676464313));
#81336=CARTESIAN_POINT('Ctrl Pts',(3.42584449768172,-0.831522847359714,
1.20719757316213));
#81337=CARTESIAN_POINT('Ctrl Pts',(3.45151131650685,-1.2185162314853,0.940652344085303));
#81338=CARTESIAN_POINT('Ctrl Pts',(3.47717813533197,-1.46476353619869,0.469724367507778));
#81339=CARTESIAN_POINT('Ctrl Pts',(3.50284495415709,-1.4658722466537,-0.00023313482661453));
#81340=CARTESIAN_POINT('Origin',(-0.510867114736157,0.,0.));
#81341=CARTESIAN_POINT('',(3.23913288526384,-1.17647078304258,-0.000815656752585949));
#81342=CARTESIAN_POINT('',(3.33786711473616,-1.17965906286054,-0.000187614992894769));
#81343=CARTESIAN_POINT('',(-0.510867114736157,-1.17775,-2.64996692395027E-14));
#81344=CARTESIAN_POINT('',(3.7365,-1.1771054344427,0.038959706177682));
#81345=CARTESIAN_POINT('Ctrl Pts',(3.23913288526384,-1.17647078304258,-0.000815656752586099));
#81346=CARTESIAN_POINT('Ctrl Pts',(3.248521940321,-1.17736613216475,-0.140117153886184));
#81347=CARTESIAN_POINT('Ctrl Pts',(3.28433506991922,-1.09011586029682,-0.670378880060937));
#81348=CARTESIAN_POINT('Ctrl Pts',(3.34657227405852,-0.30451723605224,-1.35764959839504));
#81349=CARTESIAN_POINT('Ctrl Pts',(3.42584449768172,0.973987891872518,-0.993529415162783));
#81350=CARTESIAN_POINT('Ctrl Pts',(3.50511672130493,1.36353837168639,0.277552603562025));
#81351=CARTESIAN_POINT('Ctrl Pts',(3.58438894492812,0.507782087152296,1.29539343007532));
#81352=CARTESIAN_POINT('Ctrl Pts',(3.66151670449316,-0.774995051475287,
1.13478697521395));
#81353=CARTESIAN_POINT('Ctrl Pts',(3.71222038951711,-1.16517681126,0.396292593442729));
#81354=CARTESIAN_POINT('Ctrl Pts',(3.7365,-1.17898709763096,0.0385437240067104));
#81355=CARTESIAN_POINT('',(3.7365,-0.344648939580369,1.12619366493784));
#81356=CARTESIAN_POINT('Origin',(3.7365,0.,0.));
#81357=CARTESIAN_POINT('Ctrl Pts',(3.33786711473616,-1.17965906286054,-0.000187614992895038));
#81358=CARTESIAN_POINT('Ctrl Pts',(3.3386243704521,-1.17968538668852,-0.0113456954406013));
#81359=CARTESIAN_POINT('Ctrl Pts',(3.36580570070911,-1.17446657122554,-0.411835233187));
#81360=CARTESIAN_POINT('Ctrl Pts',(3.41941110550719,-0.722370214448171,
-1.18914586543665));
#81361=CARTESIAN_POINT('Ctrl Pts',(3.49868332913039,0.60485244622559,-1.25257895798247));
#81362=CARTESIAN_POINT('Ctrl Pts',(3.57795555275359,1.38146769635508,-0.173309657930487));
#81363=CARTESIAN_POINT('Ctrl Pts',(3.6572277763768,0.893721090248042,1.06587168358242));
#81364=CARTESIAN_POINT('Ctrl Pts',(3.71007592545893,0.029308975541542,1.24063596994012));
#81365=CARTESIAN_POINT('Ctrl Pts',(3.7365,-0.344648939580369,1.12619366493784));
#81366=CARTESIAN_POINT('Origin',(-0.510867114736157,0.,0.));
#81367=CARTESIAN_POINT('',(2.73913288526384,-1.17662349254263,0.000887779294870973));
#81368=CARTESIAN_POINT('',(2.83786711473616,-1.17663586700228,-0.000891926501168649));
#81369=CARTESIAN_POINT('',(-0.510867114736157,-1.17775,-2.64996692395027E-14));
#81370=CARTESIAN_POINT('Ctrl Pts',(2.73913288526384,-1.17662349254263,0.000887779294870931));
#81371=CARTESIAN_POINT('Ctrl Pts',(2.75664415974126,-1.17479599166414,-0.258832500402587));
#81372=CARTESIAN_POINT('Ctrl Pts',(2.80057950875975,-0.96211056230301,-0.913183863350559));
#81373=CARTESIAN_POINT('Ctrl Pts',(2.87093893231929,0.118856588721082,-1.38629274593749));
#81374=CARTESIAN_POINT('Ctrl Pts',(2.9502111559425,1.22824298214487,-0.653719011308979));
#81375=CARTESIAN_POINT('Ctrl Pts',(3.0294833795657,1.21631278230501,0.675664417594188));
#81376=CARTESIAN_POINT('Ctrl Pts',(3.10875560318891,0.0939426366750465,
1.38820463693965));
#81377=CARTESIAN_POINT('Ctrl Pts',(3.17863877175495,-0.971083435973477,
0.899094198311085));
#81378=CARTESIAN_POINT('Ctrl Pts',(3.22209786577993,-1.17484630756042,0.251925828238525));
#81379=CARTESIAN_POINT('Ctrl Pts',(3.23913288526384,-1.17647078304258,-0.000815656752586099));
#81380=CARTESIAN_POINT('Ctrl Pts',(2.83786711473616,-1.17663586700228,-0.000891926501168892));
#81381=CARTESIAN_POINT('Ctrl Pts',(2.84674658987236,-1.17756805370834,-0.132585471629546));
#81382=CARTESIAN_POINT('Ctrl Pts',(2.88205013954964,-1.09646355944131,-0.655066162450786));
#81383=CARTESIAN_POINT('Ctrl Pts',(2.94377776376796,-0.330572392937332,
-1.35153966563246));
#81384=CARTESIAN_POINT('Ctrl Pts',(3.02304998739118,0.954782977733753,-1.01207480386435));
#81385=CARTESIAN_POINT('Ctrl Pts',(3.10232221101437,1.3685043706856,0.251344259488195));
#81386=CARTESIAN_POINT('Ctrl Pts',(3.18159443463759,0.532789731128058,1.28533204040039));
#81387=CARTESIAN_POINT('Ctrl Pts',(3.26010940254484,-0.776585752658408,
1.14714881787129));
#81388=CARTESIAN_POINT('Ctrl Pts',(3.31220029591104,-1.17876682935294,0.378010163192515));
#81389=CARTESIAN_POINT('Ctrl Pts',(3.33786711473616,-1.17965906286054,-0.000187614992895038));
#81390=CARTESIAN_POINT('Origin',(-0.510867114736157,0.,0.));
#81391=CARTESIAN_POINT('',(2.23913288526384,-1.17962055338313,0.000214571663858193));
#81392=CARTESIAN_POINT('',(2.33786711473616,-1.17645500278567,0.000812080812545024));
#81393=CARTESIAN_POINT('',(-0.510867114736157,-1.17775,-2.64996692395027E-14));
#81394=CARTESIAN_POINT('Ctrl Pts',(2.23913288526384,-1.17962055338313,0.000214571663858217));
#81395=CARTESIAN_POINT('Ctrl Pts',(2.26476637916152,-1.17867015320378,-0.377483674274969));
#81396=CARTESIAN_POINT('Ctrl Pts',(2.31682394760027,-0.77753452327143,-1.14626486346891));
#81397=CARTESIAN_POINT('Ctrl Pts',(2.39530559058008,0.53120860125257,-1.28598252302312));
#81398=CARTESIAN_POINT('Ctrl Pts',(2.47457781420328,1.36816948482281,-0.25307265184342));
#81399=CARTESIAN_POINT('Ctrl Pts',(2.55385003782648,0.956063119382725,1.01087931130145));
#81400=CARTESIAN_POINT('Ctrl Pts',(2.63312226144969,-0.328879200082413,
1.35195127086139));
#81401=CARTESIAN_POINT('Ctrl Pts',(2.69488321059547,-1.09605252871168,0.65606806460703));
#81402=CARTESIAN_POINT('Ctrl Pts',(2.73022008520019,-1.17755364471214,0.133078895846903));
#81403=CARTESIAN_POINT('Ctrl Pts',(2.73913288526384,-1.17662349254263,0.000887779294870931));
#81404=CARTESIAN_POINT('Ctrl Pts',(2.33786711473616,-1.17645500278567,0.00081208081254492));
#81405=CARTESIAN_POINT('Ctrl Pts',(2.35486880929262,-1.17484701827737,-0.251441262450268));
#81406=CARTESIAN_POINT('Ctrl Pts',(2.39829457839015,-0.971713036485233,
-0.898110065252741));
#81407=CARTESIAN_POINT('Ctrl Pts',(2.46814442202875,0.0922039693498821,
-1.3883200119834));
#81408=CARTESIAN_POINT('Ctrl Pts',(2.54741664565196,1.21546005757808,-0.677192797651213));
#81409=CARTESIAN_POINT('Ctrl Pts',(2.62668886927516,1.22906522301855,0.65217574590713));
#81410=CARTESIAN_POINT('Ctrl Pts',(2.70596109289836,0.120596640913772,1.38614255166615));
#81411=CARTESIAN_POINT('Ctrl Pts',(2.77635384138536,-0.96147348091212,0.914167980049009));
#81412=CARTESIAN_POINT('Ctrl Pts',(2.82032251533129,-1.1747939966127,0.259316076566906));
#81413=CARTESIAN_POINT('Ctrl Pts',(2.83786711473616,-1.17663586700228,-0.000891926501168892));
#81414=CARTESIAN_POINT('Origin',(-0.510867114736157,0.,0.));
#81415=CARTESIAN_POINT('',(1.73913288526384,-1.17723576271456,-0.00104224624287887));
#81416=CARTESIAN_POINT('',(1.83786711473616,-1.17954252137753,0.000348062568210376));
#81417=CARTESIAN_POINT('',(-0.510867114736157,-1.17775,-2.64996692395027E-14));
#81418=CARTESIAN_POINT('Ctrl Pts',(1.73913288526384,-1.17723576271456,-0.00104224624287901));
#81419=CARTESIAN_POINT('Ctrl Pts',(1.74646452404071,-1.17816845504985,-0.109639245293173));
#81420=CARTESIAN_POINT('Ctrl Pts',(1.78022023735865,-1.11464558726191,-0.608561633391758));
#81421=CARTESIAN_POINT('Ctrl Pts',(1.84040002521766,-0.408834878719842,
-1.32995772423544));
#81422=CARTESIAN_POINT('Ctrl Pts',(1.91967224884086,0.894143840963125,-1.06603959552792));
#81423=CARTESIAN_POINT('Ctrl Pts',(1.99894447246406,1.3808158933056,0.17111712463292));
#81424=CARTESIAN_POINT('Ctrl Pts',(2.07821669608726,0.606875073722467,1.2520528059251));
#81425=CARTESIAN_POINT('Ctrl Pts',(2.15748891971047,-0.721111027024888,
1.18992961688625));
#81426=CARTESIAN_POINT('Ctrl Pts',(2.21112764943599,-1.17422232882441,0.41283140296388));
#81427=CARTESIAN_POINT('Ctrl Pts',(2.23834230462045,-1.17964986534459,0.0118634293448927));
#81428=CARTESIAN_POINT('Ctrl Pts',(2.23913288526384,-1.17962055338313,0.000214571663858217));
#81429=CARTESIAN_POINT('Ctrl Pts',(1.83786711473616,-1.17954252137753,0.000348062568210372));
#81430=CARTESIAN_POINT('Ctrl Pts',(1.86299102871288,-1.17809536271031,-0.369907373018322));
#81431=CARTESIAN_POINT('Ctrl Pts',(1.91453901723068,-0.790931654118442,
-1.13218761048638));
#81432=CARTESIAN_POINT('Ctrl Pts',(1.99251108028953,0.506407483735447,-1.29594958554484));
#81433=CARTESIAN_POINT('Ctrl Pts',(2.07178330391274,1.3630557428063,-0.279307872204986));
#81434=CARTESIAN_POINT('Ctrl Pts',(2.15105552753594,0.975305236911186,0.992327344111197));
#81435=CARTESIAN_POINT('Ctrl Pts',(2.23032775115914,-0.302848092395607,
1.35801948506016));
#81436=CARTESIAN_POINT('Ctrl Pts',(2.29259828022588,-1.08968667651,0.671382772571054));
#81437=CARTESIAN_POINT('Ctrl Pts',(2.32844473475155,-1.17734615166475,0.140611489907658));
#81438=CARTESIAN_POINT('Ctrl Pts',(2.33786711473616,-1.17645500278567,0.00081208081254492));
#81439=CARTESIAN_POINT('Origin',(-0.510867114736157,0.,0.));
#81440=CARTESIAN_POINT('',(1.23913288526384,-1.17605505019199,0.000522350384450236));
#81441=CARTESIAN_POINT('',(1.33786711473616,-1.1774542148928,-0.00106316141115878));
#81442=CARTESIAN_POINT('',(-0.510867114736157,-1.17775,-2.64996692395027E-14));
#81443=CARTESIAN_POINT('Ctrl Pts',(1.23913288526384,-1.17605505019199,0.000522350384450018));
#81444=CARTESIAN_POINT('Ctrl Pts',(1.25458674346097,-1.17513676588396,-0.22896185759751));
#81445=CARTESIAN_POINT('Ctrl Pts',(1.29646467619917,-0.999534094584203,
-0.852133676211331));
#81446=CARTESIAN_POINT('Ctrl Pts',(1.36476668347844,0.0110818382145732,
-1.39133265677073));
#81447=CARTESIAN_POINT('Ctrl Pts',(1.44403890710164,1.1738981497851,-0.746925431386865));
#81448=CARTESIAN_POINT('Ctrl Pts',(1.52331113072484,1.26500718194706,0.579388553442205));
#81449=CARTESIAN_POINT('Ctrl Pts',(1.60258335434805,0.201230401682631,1.37674954089208));
#81450=CARTESIAN_POINT('Ctrl Pts',(1.67452393919438,-0.930882719706594,
0.959712096433582));
#81451=CARTESIAN_POINT('Ctrl Pts',(1.72004044949964,-1.17480692394588,0.281756905713905));
#81452=CARTESIAN_POINT('Ctrl Pts',(1.73913288526384,-1.17723576271456,-0.00104224624287901));
#81453=CARTESIAN_POINT('Ctrl Pts',(1.33786711473616,-1.1774542148928,-0.00106316141115873));
#81454=CARTESIAN_POINT('Ctrl Pts',(1.34468917359208,-1.17835294650458,-0.102064601296605));
#81455=CARTESIAN_POINT('Ctrl Pts',(1.37793530698906,-1.12027215618224,-0.593259967820105));
#81456=CARTESIAN_POINT('Ctrl Pts',(1.43760551492711,-0.434307261820031,
-1.32185870617429));
#81457=CARTESIAN_POINT('Ctrl Pts',(1.51687773855032,0.873500757568272,-1.08301913841129));
#81458=CARTESIAN_POINT('Ctrl Pts',(1.59614996217352,1.38384829755233,0.144560786138938));
#81459=CARTESIAN_POINT('Ctrl Pts',(1.67542218579672,0.630814469109849,1.24016405114351));
#81460=CARTESIAN_POINT('Ctrl Pts',(1.75469440941992,-0.698120020172913,
1.20356234832455));
#81461=CARTESIAN_POINT('Ctrl Pts',(1.8088427190664,-1.17052112656004,0.428012959930639));
#81462=CARTESIAN_POINT('Ctrl Pts',(1.83656695417181,-1.17961741172428,0.0195087521219825));
#81463=CARTESIAN_POINT('Ctrl Pts',(1.83786711473616,-1.17954252137753,0.000348062568210372));
#81464=CARTESIAN_POINT('Origin',(-0.510867114736157,0.,0.));
#81465=CARTESIAN_POINT('',(0.739132885263843,-1.17911213255423,0.000786107540026912));
#81466=CARTESIAN_POINT('',(0.837867114736159,-1.17596232425638,0.000418044704970089));
#81467=CARTESIAN_POINT('',(-0.510867114736157,-1.17775,-2.64996692395027E-14));
#81468=CARTESIAN_POINT('Ctrl Pts',(0.739132885263843,-1.17911213255423,
0.000786107540026912));
#81469=CARTESIAN_POINT('Ctrl Pts',(0.762708962881233,-1.17664592192968,
-0.346963469627478));
#81470=CARTESIAN_POINT('Ctrl Pts',(0.812709115039692,-0.830115587406687,
-1.08901150369434));
#81471=CARTESIAN_POINT('Ctrl Pts',(0.889133341739219,0.429979607970486,
-1.32320468901736));
#81472=CARTESIAN_POINT('Ctrl Pts',(0.968405565362423,1.34444024085867,-0.358362411303147));
#81473=CARTESIAN_POINT('Ctrl Pts',(1.04767778898562,1.03152012276366,0.933779522210948));
#81474=CARTESIAN_POINT('Ctrl Pts',(1.12695001260883,-0.223136159389758,
1.3733593350842));
#81475=CARTESIAN_POINT('Ctrl Pts',(1.1907683780349,-1.06919746578618,0.717893990913368));
#81476=CARTESIAN_POINT('Ctrl Pts',(1.2281626689199,-1.17670691184336,0.16342609758892));
#81477=CARTESIAN_POINT('Ctrl Pts',(1.23913288526384,-1.17605505019199,0.000522350384450018));
#81478=CARTESIAN_POINT('Ctrl Pts',(0.837867114736159,-1.17596232425638,
0.000418044704970002));
#81479=CARTESIAN_POINT('Ctrl Pts',(0.852811393012336,-1.17526879968713,
-0.221545053987815));
#81480=CARTESIAN_POINT('Ctrl Pts',(0.89417974582958,-1.00826246762855,-0.836955378552283));
#81481=CARTESIAN_POINT('Ctrl Pts',(0.961972173187893,-0.0156437653744218,
-1.39128042313263));
#81482=CARTESIAN_POINT('Ctrl Pts',(1.0412443968111,1.15933180789216,-0.769342143626431));
#81483=CARTESIAN_POINT('Ctrl Pts',(1.1205166204343,1.27590453729514,0.554983829328479));
#81484=CARTESIAN_POINT('Ctrl Pts',(1.1997888440575,0.227639519397196,1.3726288257033));
#81485=CARTESIAN_POINT('Ctrl Pts',(1.27223900882479,-0.920349622811229,
0.974617948196986));
#81486=CARTESIAN_POINT('Ctrl Pts',(1.31826509905101,-1.17487186379867,0.289147147627791));
#81487=CARTESIAN_POINT('Ctrl Pts',(1.33786711473616,-1.1774542148928,-0.00106316141115873));
#81488=CARTESIAN_POINT('Origin',(3.7365,3.28582941601228E-17,0.));
#81489=CARTESIAN_POINT('',(3.7365,0.66187319412785,-1.30528009442227));
#81490=CARTESIAN_POINT('Ctrl Pts',(3.7365,-1.17898709763096,0.0385437240067023));
#81491=CARTESIAN_POINT('Ctrl Pts',(3.7365,-1.18395318976076,0.0068885070196644));
#81492=CARTESIAN_POINT('Ctrl Pts',(3.7365,-1.18753666953077,-0.0249123100679694));
#81493=CARTESIAN_POINT('Ctrl Pts',(3.7365,-1.1896998725534,-0.0567807570343834));
#81494=CARTESIAN_POINT('Ctrl Pts',(3.7365,-1.19296909471786,-0.104943149597595));
#81495=CARTESIAN_POINT('Ctrl Pts',(3.7365,-1.19299730966002,-0.153259572705676));
#81496=CARTESIAN_POINT('Ctrl Pts',(3.7365,-1.18997678969837,-0.201492670338683));
#81497=CARTESIAN_POINT('Ctrl Pts',(3.7365,-1.18852496860528,-0.224676039234535));
#81498=CARTESIAN_POINT('Ctrl Pts',(3.7365,-1.18636806011878,-0.247840396141398));
#81499=CARTESIAN_POINT('Ctrl Pts',(3.7365,-1.18352338482475,-0.270960259527509));
#81500=CARTESIAN_POINT('Ctrl Pts',(3.7365,-1.18229282775955,-0.28096151038943));
#81501=CARTESIAN_POINT('Ctrl Pts',(3.7365,-1.18093363039742,-0.290953014018376));
#81502=CARTESIAN_POINT('Ctrl Pts',(3.7365,-1.17944884835669,-0.300923054854913));
#81503=CARTESIAN_POINT('Ctrl Pts',(3.7365,-1.17199727383116,-0.350959019917949));
#81504=CARTESIAN_POINT('Ctrl Pts',(3.7365,-1.16137910126565,-0.400519951283811));
#81505=CARTESIAN_POINT('Ctrl Pts',(3.7365,-1.14780434654206,-0.449345351076564));
#81506=CARTESIAN_POINT('Ctrl Pts',(3.7365,-1.1381603195141,-0.484032789990987));
#81507=CARTESIAN_POINT('Ctrl Pts',(3.7365,-1.12702287204522,-0.518349414699403));
#81508=CARTESIAN_POINT('Ctrl Pts',(3.7365,-1.11445155766447,-0.552203463055681));
#81509=CARTESIAN_POINT('Ctrl Pts',(3.7365,-1.10956752286223,-0.565355974031146));
#81510=CARTESIAN_POINT('Ctrl Pts',(3.7365,-1.10446693006086,-0.578438661643457));
#81511=CARTESIAN_POINT('Ctrl Pts',(3.7365,-1.09915277069566,-0.591446096472848));
#81512=CARTESIAN_POINT('Ctrl Pts',(3.7365,-1.09531873084628,-0.600830651968257));
#81513=CARTESIAN_POINT('Ctrl Pts',(3.7365,-1.09137504997109,-0.610172118209165));
#81514=CARTESIAN_POINT('Ctrl Pts',(3.7365,-1.087326496467,-0.619461079847843));
#81515=CARTESIAN_POINT('Ctrl Pts',(3.7365,-1.06633587924426,-0.667621747097829));
#81516=CARTESIAN_POINT('Ctrl Pts',(3.7365,-1.04250587869293,-0.714431076751343));
#81517=CARTESIAN_POINT('Ctrl Pts',(3.7365,-1.01604654267101,-0.75962191442263));
#81518=CARTESIAN_POINT('Ctrl Pts',(3.7365,-0.989101302874277,-0.805642644370617));
#81519=CARTESIAN_POINT('Ctrl Pts',(3.7365,-0.959429029561841,-0.849986048299225));
#81520=CARTESIAN_POINT('Ctrl Pts',(3.7365,-0.927198803465423,-0.892364654491487));
#81521=CARTESIAN_POINT('Ctrl Pts',(3.7365,-0.908698673052218,-0.916689948981861));
#81522=CARTESIAN_POINT('Ctrl Pts',(3.7365,-0.889354812189278,-0.940367701839285));
#81523=CARTESIAN_POINT('Ctrl Pts',(3.7365,-0.869192074342517,-0.963340448953061));
#81524=CARTESIAN_POINT('Ctrl Pts',(3.7365,-0.857848710493305,-0.976264697192959));
#81525=CARTESIAN_POINT('Ctrl Pts',(3.7365,-0.846246075599409,-0.988965753946543));
#81526=CARTESIAN_POINT('Ctrl Pts',(3.7365,-0.834387932224055,-1.00143289879475));
#81527=CARTESIAN_POINT('Ctrl Pts',(3.7365,-0.827553225622948,-1.00861861703864));
#81528=CARTESIAN_POINT('Ctrl Pts',(3.7365,-0.820633298378763,-1.01572679588455));
#81529=CARTESIAN_POINT('Ctrl Pts',(3.7365,-0.813639868172984,-1.02274468687781));
#81530=CARTESIAN_POINT('Ctrl Pts',(3.7365,-0.774949026471088,-1.06157085679896));
#81531=CARTESIAN_POINT('Ctrl Pts',(3.7365,-0.733934919892263,-1.09771763061715));
#81532=CARTESIAN_POINT('Ctrl Pts',(3.7365,-0.69079018012452,-1.13089396681559));
#81533=CARTESIAN_POINT('Ctrl Pts',(3.7365,-0.683113793755067,-1.13679675766224));
#81534=CARTESIAN_POINT('Ctrl Pts',(3.7365,-0.675369835460676,-1.14260546817357));
#81535=CARTESIAN_POINT('Ctrl Pts',(3.7365,-0.667559232793028,-1.14831838686635));
#81536=CARTESIAN_POINT('Ctrl Pts',(3.7365,-0.625187949984191,-1.17931006624061));
#81537=CARTESIAN_POINT('Ctrl Pts',(3.7365,-0.580858497988276,-1.20748566736297));
#81538=CARTESIAN_POINT('Ctrl Pts',(3.7365,-0.534866759029188,-1.23287345299529));
#81539=CARTESIAN_POINT('Ctrl Pts',(3.7365,-0.511266715166499,-1.24590085461261));
#81540=CARTESIAN_POINT('Ctrl Pts',(3.7365,-0.48722834897051,-1.25819361049471));
#81541=CARTESIAN_POINT('Ctrl Pts',(3.7365,-0.462788279793142,-1.26975163493864));
#81542=CARTESIAN_POINT('Ctrl Pts',(3.7365,-0.447910497377259,-1.27678753044231));
#81543=CARTESIAN_POINT('Ctrl Pts',(3.7365,-0.432883815548152,-1.28355110292038));
#81544=CARTESIAN_POINT('Ctrl Pts',(3.7365,-0.41771617777022,-1.29004182329204));
#81545=CARTESIAN_POINT('Ctrl Pts',(3.7365,-0.407705569003771,-1.29432568497205));
#81546=CARTESIAN_POINT('Ctrl Pts',(3.7365,-0.397632108665662,-1.2984911384465));
#81547=CARTESIAN_POINT('Ctrl Pts',(3.7365,-0.38751563048501,-1.30253128217036));
#81548=CARTESIAN_POINT('Ctrl Pts',(3.7365,-0.336601391291811,-1.32286452860831));
#81549=CARTESIAN_POINT('Ctrl Pts',(3.7365,-0.284504357316613,-1.34006945525572));
#81550=CARTESIAN_POINT('Ctrl Pts',(3.7365,-0.231557314522765,-1.35419331042861));
#81551=CARTESIAN_POINT('Ctrl Pts',(3.7365,-0.177455970281344,-1.36862508055975));
#81552=CARTESIAN_POINT('Ctrl Pts',(3.7365,-0.12246626002564,-1.37984038062529));
#81553=CARTESIAN_POINT('Ctrl Pts',(3.7365,-0.066909525356045,-1.38784621613597));
#81554=CARTESIAN_POINT('Ctrl Pts',(3.7365,-0.0356886580014238,-1.39234520496295));
#81555=CARTESIAN_POINT('Ctrl Pts',(3.7365,-0.00428819436563625,-1.39582982383752));
#81556=CARTESIAN_POINT('Ctrl Pts',(3.7365,0.0272376679168194,-1.39829475873246));
#81557=CARTESIAN_POINT('Ctrl Pts',(3.7365,0.047886366616149,-1.39990923314407));
#81558=CARTESIAN_POINT('Ctrl Pts',(3.7365,0.0685888961784583,-1.40108617121842));
#81559=CARTESIAN_POINT('Ctrl Pts',(3.7365,0.0893302635243502,-1.40182292113385));
#81560=CARTESIAN_POINT('Ctrl Pts',(3.7365,0.0997890716871271,-1.40219442634375));
#81561=CARTESIAN_POINT('Ctrl Pts',(3.7365,0.11026029244007,-1.40245402241009));
#81562=CARTESIAN_POINT('Ctrl Pts',(3.7365,0.120733734333452,-1.40260117612064));
#81563=CARTESIAN_POINT('Ctrl Pts',(3.7365,0.178939128318525,-1.40341897219821));
#81564=CARTESIAN_POINT('Ctrl Pts',(3.7365,0.237032745754499,-1.40076707020305));
#81565=CARTESIAN_POINT('Ctrl Pts',(3.7365,0.294671049963821,-1.39466962302802));
#81566=CARTESIAN_POINT('Ctrl Pts',(3.7365,0.35245700073739,-1.38855655660224));
#81567=CARTESIAN_POINT('Ctrl Pts',(3.7365,0.409786446730489,-1.37898053666939));
#81568=CARTESIAN_POINT('Ctrl Pts',(3.7365,0.466329084911745,-1.36591626968488));
#81569=CARTESIAN_POINT('Ctrl Pts',(3.7365,0.521568448510678,-1.35315312637705));
#81570=CARTESIAN_POINT('Ctrl Pts',(3.7365,0.576057945793192,-1.33706073718071));
#81571=CARTESIAN_POINT('Ctrl Pts',(3.7365,0.629488202861402,-1.31756621599704));
#81572=CARTESIAN_POINT('Ctrl Pts',(3.7365,0.640327714531275,-1.31361132037302));
#81573=CARTESIAN_POINT('Ctrl Pts',(3.7365,0.651123595619572,-1.30951623562727));
#81574=CARTESIAN_POINT('Ctrl Pts',(3.7365,0.661873194127841,-1.30528009442227));
#81575=CARTESIAN_POINT('',(3.7365,-1.4635,-1.79227059055215E-16));
#81576=CARTESIAN_POINT('Origin',(3.7365,0.,0.));
#81577=CARTESIAN_POINT('',(3.7365,1.43393351041226,-0.298434655783759));
#81578=CARTESIAN_POINT('Origin',(3.7365,0.,0.));
#81579=CARTESIAN_POINT('Ctrl Pts',(3.7365,1.43512958320548,-0.29838030867993));
#81580=CARTESIAN_POINT('Ctrl Pts',(3.7365,1.43970072126023,-0.259303035834852));
#81581=CARTESIAN_POINT('Ctrl Pts',(3.7365,1.44258412773515,-0.22010113429756));
#81582=CARTESIAN_POINT('Ctrl Pts',(3.7365,1.44371345760419,-0.180852703561548));
#81583=CARTESIAN_POINT('Ctrl Pts',(3.7365,1.44536844720772,-0.123335633834173));
#81584=CARTESIAN_POINT('Ctrl Pts',(3.7365,1.44325833111679,-0.0657175785747762));
#81585=CARTESIAN_POINT('Ctrl Pts',(3.7365,1.43753775138039,-0.00830635976255858));
#81586=CARTESIAN_POINT('Ctrl Pts',(3.7365,1.43561812626606,0.0109588235850785));
#81587=CARTESIAN_POINT('Ctrl Pts',(3.7365,1.43329155082908,0.0302005775953646));
#81588=CARTESIAN_POINT('Ctrl Pts',(3.7365,1.43056272371359,0.0494067470887997));
#81589=CARTESIAN_POINT('Ctrl Pts',(3.7365,1.42888893925048,0.0611872618423588));
#81590=CARTESIAN_POINT('Ctrl Pts',(3.7365,1.42706380724748,0.0729543826609247));
#81591=CARTESIAN_POINT('Ctrl Pts',(3.7365,1.42508831579175,0.0847052377538888));
#81592=CARTESIAN_POINT('Ctrl Pts',(3.7365,1.42299842767926,0.0971365607541427));
#81593=CARTESIAN_POINT('Ctrl Pts',(3.7365,1.4207417497427,0.109540674919579));
#81594=CARTESIAN_POINT('Ctrl Pts',(3.7365,1.41832075091978,0.121911261685987));
#81595=CARTESIAN_POINT('Ctrl Pts',(3.7365,1.40726488370833,0.178403467845804));
#81596=CARTESIAN_POINT('Ctrl Pts',(3.7365,1.39278238314873,0.234219775072268));
#81597=CARTESIAN_POINT('Ctrl Pts',(3.7365,1.3750275593212,0.289049165597431));
#81598=CARTESIAN_POINT('Ctrl Pts',(3.7365,1.36331774565455,0.325210715424246));
#81599=CARTESIAN_POINT('Ctrl Pts',(3.7365,1.35018350192035,0.360942623635693));
#81600=CARTESIAN_POINT('Ctrl Pts',(3.7365,1.33565892575706,0.396148542417578));
#81601=CARTESIAN_POINT('Ctrl Pts',(3.7365,1.33049266787634,0.408670963265526));
#81602=CARTESIAN_POINT('Ctrl Pts',(3.7365,1.32515044411142,0.421126773855556));
#81603=CARTESIAN_POINT('Ctrl Pts',(3.7365,1.31963357868943,0.433511409073657));
#81604=CARTESIAN_POINT('Ctrl Pts',(3.7365,1.31439779966332,0.445265042407288));
#81605=CARTESIAN_POINT('Ctrl Pts',(3.7365,1.3090038207151,0.456956118390431));
#81606=CARTESIAN_POINT('Ctrl Pts',(3.7365,1.30346243158798,0.468561223712885));
#81607=CARTESIAN_POINT('Ctrl Pts',(3.7365,1.27922239399636,0.519326146157052));
#81608=CARTESIAN_POINT('Ctrl Pts',(3.7365,1.2521280954727,0.568534300549584));
#81609=CARTESIAN_POINT('Ctrl Pts',(3.7365,1.22232167814254,0.615895849808824));
#81610=CARTESIAN_POINT('Ctrl Pts',(3.7365,1.19326257719367,0.662069934596494));
#81611=CARTESIAN_POINT('Ctrl Pts',(3.7365,1.16162489851506,0.706489580149001));
#81612=CARTESIAN_POINT('Ctrl Pts',(3.7365,1.12750665010922,0.74885119383388));
#81613=CARTESIAN_POINT('Ctrl Pts',(3.7365,1.10741856610523,0.773792792362729));
#81614=CARTESIAN_POINT('Ctrl Pts',(3.7365,1.08646998561998,0.798020235695572));
#81615=CARTESIAN_POINT('Ctrl Pts',(3.7365,1.06467675390854,0.821464153697248));
#81616=CARTESIAN_POINT('Ctrl Pts',(3.7365,1.04901069950777,0.838316803164048));
#81617=CARTESIAN_POINT('Ctrl Pts',(3.7365,1.03290811296377,0.854764454447756));
#81618=CARTESIAN_POINT('Ctrl Pts',(3.7365,1.01637411063827,0.870779272925361));
#81619=CARTESIAN_POINT('Ctrl Pts',(3.7365,1.00938013201465,0.877553633778137));
#81620=CARTESIAN_POINT('Ctrl Pts',(3.7365,1.00230930693102,0.884250039088091));
#81621=CARTESIAN_POINT('Ctrl Pts',(3.7365,0.995171997621989,0.890857486243074));
#81622=CARTESIAN_POINT('Ctrl Pts',(3.7365,0.956476284193968,0.926680493279688));
#81623=CARTESIAN_POINT('Ctrl Pts',(3.7365,0.915755145653486,0.959964172630004));
#81624=CARTESIAN_POINT('Ctrl Pts',(3.7365,0.873106335678439,0.990433823056644));
#81625=CARTESIAN_POINT('Ctrl Pts',(3.7365,0.864608521552303,0.996504928580231));
#81626=CARTESIAN_POINT('Ctrl Pts',(3.7365,0.856034094162739,1.00246417157846));
#81627=CARTESIAN_POINT('Ctrl Pts',(3.7365,0.847383710313845,1.00830915591921));
#81628=CARTESIAN_POINT('Ctrl Pts',(3.7365,0.800817662288227,1.0397734037809));
#81629=CARTESIAN_POINT('Ctrl Pts',(3.7365,0.752051536069289,1.06793166378029));
#81630=CARTESIAN_POINT('Ctrl Pts',(3.7365,0.701457004762612,1.09273173067751));
#81631=CARTESIAN_POINT('Ctrl Pts',(3.7365,0.679744688332938,1.10337451925649));
#81632=CARTESIAN_POINT('Ctrl Pts',(3.7365,0.657695506324503,1.1133980690338));
#81633=CARTESIAN_POINT('Ctrl Pts',(3.7365,0.63533868558444,1.12279473411649));
#81634=CARTESIAN_POINT('Ctrl Pts',(3.7365,0.619306521374032,1.12953311965831));
#81635=CARTESIAN_POINT('Ctrl Pts',(3.7365,0.603116157757065,1.13594909322168));
#81636=CARTESIAN_POINT('Ctrl Pts',(3.7365,0.586778487209965,1.14203916526268));
#81637=CARTESIAN_POINT('Ctrl Pts',(3.7365,0.577296942343772,1.14557353028299));
#81638=CARTESIAN_POINT('Ctrl Pts',(3.7365,0.567774044499413,1.14899500605876));
#81639=CARTESIAN_POINT('Ctrl Pts',(3.7365,0.558216209668818,1.15230211828721));
#81640=CARTESIAN_POINT('Ctrl Pts',(3.7365,0.508587976552736,1.16947401333705));
#81641=CARTESIAN_POINT('Ctrl Pts',(3.7365,0.457982493420678,1.1835801791689));
#81642=CARTESIAN_POINT('Ctrl Pts',(3.7365,0.406709608338887,1.1946002349887));
#81643=CARTESIAN_POINT('Ctrl Pts',(3.7365,0.355691719174312,1.2055654846622));
#81644=CARTESIAN_POINT('Ctrl Pts',(3.7365,0.304011857242369,1.21347515766827));
#81645=CARTESIAN_POINT('Ctrl Pts',(3.7365,0.251977513100709,1.21825818903545));
#81646=CARTESIAN_POINT('Ctrl Pts',(3.7365,0.225944148236759,1.2206511931713));
#81647=CARTESIAN_POINT('Ctrl Pts',(3.7365,0.199822199175476,1.2222607723633));
#81648=CARTESIAN_POINT('Ctrl Pts',(3.7365,0.173651787414364,1.2230732991355));
#81649=CARTESIAN_POINT('Ctrl Pts',(3.7365,0.154357834140816,1.2236723288229));
#81650=CARTESIAN_POINT('Ctrl Pts',(3.7365,0.135037563201662,1.2238380736161));
#81651=CARTESIAN_POINT('Ctrl Pts',(3.7365,0.1157076553361,1.22356398342678));
#81652=CARTESIAN_POINT('Ctrl Pts',(3.7365,0.106361568937003,1.22343145974336));
#81653=CARTESIAN_POINT('Ctrl Pts',(3.7365,0.0970142683297624,1.22319601976542));
#81654=CARTESIAN_POINT('Ctrl Pts',(3.7365,0.0876804416350563,1.22285765921622));
#81655=CARTESIAN_POINT('Ctrl Pts',(3.7365,0.0372834290399511,1.2210307171251));
#81656=CARTESIAN_POINT('Ctrl Pts',(3.7365,-0.0128221292937848,1.2162064058474));
#81657=CARTESIAN_POINT('Ctrl Pts',(3.7365,-0.0623571086805372,1.20833476103376));
#81658=CARTESIAN_POINT('Ctrl Pts',(3.7365,-0.110880903841195,1.20062380434732));
#81659=CARTESIAN_POINT('Ctrl Pts',(3.7365,-0.15885808999604,1.18998841684919));
#81660=CARTESIAN_POINT('Ctrl Pts',(3.7365,-0.206006127539271,1.17633630959573));
#81661=CARTESIAN_POINT('Ctrl Pts',(3.7365,-0.253154165082502,1.16268420234226));
#81662=CARTESIAN_POINT('Ctrl Pts',(3.7365,-0.299473974845737,1.14601529259411));
#81663=CARTESIAN_POINT('Ctrl Pts',(3.7365,-0.344648939580368,1.12619366493784));
#81664=CARTESIAN_POINT('Ctrl Pts',(0.248522160579065,-0.510216505388422,
1.06149619882938));
#81665=CARTESIAN_POINT('Ctrl Pts',(0.274946235120132,-0.862691321916517,
0.892076403144088));
#81666=CARTESIAN_POINT('Ctrl Pts',(0.327794384202268,-1.37960057435709,
0.177544609184711));
#81667=CARTESIAN_POINT('Ctrl Pts',(0.407066607825471,-0.89796482962545,
-1.06402462300472));
#81668=CARTESIAN_POINT('Ctrl Pts',(0.486338831448674,0.404638909243713,
-1.33081474323498));
#81669=CARTESIAN_POINT('Ctrl Pts',(0.565611055071876,1.33722609341091,-0.384334478167097));
#81670=CARTESIAN_POINT('Ctrl Pts',(0.644883278695081,1.0493104811472,0.913903580847046));
#81671=CARTESIAN_POINT('Ctrl Pts',(0.724155502318283,-0.196736085198769,
1.37733389209964));
#81672=CARTESIAN_POINT('Ctrl Pts',(0.803427725941487,-1.26308608578749,
0.583572524683419));
#81673=CARTESIAN_POINT('Ctrl Pts',(0.882699949564689,-1.17634997997517,
-0.743087393228864));
#81674=CARTESIAN_POINT('Ctrl Pts',(0.961972173187893,-0.0156437653744218,
-1.39128042313263));
#81675=CARTESIAN_POINT('Ctrl Pts',(1.0412443968111,1.15933180789216,-0.769342143626431));
#81676=CARTESIAN_POINT('Ctrl Pts',(1.1205166204343,1.27590453729514,0.554983829328479));
#81677=CARTESIAN_POINT('Ctrl Pts',(1.1997888440575,0.227639519397196,1.3726288257033));
#81678=CARTESIAN_POINT('Ctrl Pts',(1.2790610676807,-1.02844667848052,0.937140412564534));
#81679=CARTESIAN_POINT('Ctrl Pts',(1.35833329130391,-1.34561567488944,-0.353910979590878));
#81680=CARTESIAN_POINT('Ctrl Pts',(1.43760551492711,-0.434307261820031,
-1.32185870617429));
#81681=CARTESIAN_POINT('Ctrl Pts',(1.51687773855032,0.873500757568272,-1.08301913841129));
#81682=CARTESIAN_POINT('Ctrl Pts',(1.59614996217352,1.38384829755233,0.144560786138938));
#81683=CARTESIAN_POINT('Ctrl Pts',(1.67542218579672,0.630814469109849,1.24016405114351));
#81684=CARTESIAN_POINT('Ctrl Pts',(1.75469440941992,-0.698120020172913,
1.20356234832455));
#81685=CARTESIAN_POINT('Ctrl Pts',(1.83396663304313,-1.38970737331209,0.0681709584735189));
#81686=CARTESIAN_POINT('Ctrl Pts',(1.91323885666633,-0.812564391786863,
-1.12945692909156));
#81687=CARTESIAN_POINT('Ctrl Pts',(1.99251108028953,0.506407483735447,-1.29594958554484));
#81688=CARTESIAN_POINT('Ctrl Pts',(2.07178330391274,1.3630557428063,-0.279307872204986));
#81689=CARTESIAN_POINT('Ctrl Pts',(2.15105552753594,0.975305236911186,0.992327344111197));
#81690=CARTESIAN_POINT('Ctrl Pts',(2.23032775115914,-0.302848092395607,
1.35801948506016));
#81691=CARTESIAN_POINT('Ctrl Pts',(2.30959997478234,-1.30451686139594,0.48391065964775));
#81692=CARTESIAN_POINT('Ctrl Pts',(2.38887219840555,-1.11522989749538,-0.831983297464578));
#81693=CARTESIAN_POINT('Ctrl Pts',(2.46814442202875,0.0922039693498821,
-1.3883200119834));
#81694=CARTESIAN_POINT('Ctrl Pts',(2.54741664565196,1.21546005757808,-0.677192797651213));
#81695=CARTESIAN_POINT('Ctrl Pts',(2.62668886927516,1.22906522301855,0.65217574590713));
#81696=CARTESIAN_POINT('Ctrl Pts',(2.70596109289836,0.120596640913772,1.38614255166615));
#81697=CARTESIAN_POINT('Ctrl Pts',(2.78523331652156,-1.09796786348556,0.854632210191007));
#81698=CARTESIAN_POINT('Ctrl Pts',(2.86450554014477,-1.31414978783895,-0.457110242971296));
#81699=CARTESIAN_POINT('Ctrl Pts',(2.94377776376796,-0.330572392937332,
-1.35153966563246));
#81700=CARTESIAN_POINT('Ctrl Pts',(3.02304998739118,0.954782977733753,-1.01207480386435));
#81701=CARTESIAN_POINT('Ctrl Pts',(3.10232221101437,1.3685043706856,0.251344259488195));
#81702=CARTESIAN_POINT('Ctrl Pts',(3.18159443463759,0.532789731128058,1.28533204040039));
#81703=CARTESIAN_POINT('Ctrl Pts',(3.26086665826078,-0.789214326493944,
1.14581607791232));
#81704=CARTESIAN_POINT('Ctrl Pts',(3.34013888188399,-1.39093495393087,-0.0396509125210518));
#81705=CARTESIAN_POINT('Ctrl Pts',(3.41941110550719,-0.722370214448171,
-1.18914586543665));
#81706=CARTESIAN_POINT('Ctrl Pts',(3.49868332913039,0.60485244622559,-1.25257895798247));
#81707=CARTESIAN_POINT('Ctrl Pts',(3.57795555275359,1.38146769635508,-0.173309657930487));
#81708=CARTESIAN_POINT('Ctrl Pts',(3.6572277763768,0.893721090248042,1.06587168358242));
#81709=CARTESIAN_POINT('Ctrl Pts',(3.71007592545893,0.029308975541542,1.24063596994012));
#81710=CARTESIAN_POINT('Ctrl Pts',(3.7365,-0.344648939580369,1.12619366493784));
#81711=CARTESIAN_POINT('Ctrl Pts',(0.303514773719376,-0.55148003511735,
1.14734422509854));
#81712=CARTESIAN_POINT('Ctrl Pts',(0.329938848260444,-0.932461093440649,
0.964222679857717));
#81713=CARTESIAN_POINT('Ctrl Pts',(0.38278699734258,-1.49117514850909,0.191903449367132));
#81714=CARTESIAN_POINT('Ctrl Pts',(0.462059220965783,-0.970587330174655,
-1.15007713443856));
#81715=CARTESIAN_POINT('Ctrl Pts',(0.541331444588985,0.437363898507531,
-1.4384437853009));
#81716=CARTESIAN_POINT('Ctrl Pts',(0.620603668212189,1.44537365053032,-0.415417355726357));
#81717=CARTESIAN_POINT('Ctrl Pts',(0.699875891835392,1.13417299299545,0.98781512071177));
#81718=CARTESIAN_POINT('Ctrl Pts',(0.779148115458594,-0.212647027347087,
1.4887251493465));
#81719=CARTESIAN_POINT('Ctrl Pts',(0.8584203390818,-1.36523760323283,0.630768689383992));
#81720=CARTESIAN_POINT('Ctrl Pts',(0.937692562705,-1.27148675398718,-0.803184250970361));
#81721=CARTESIAN_POINT('Ctrl Pts',(1.01696478632821,-0.016908947842616,
-1.50379959978589));
#81722=CARTESIAN_POINT('Ctrl Pts',(1.09623700995141,1.25309224491337,-0.831562342463553));
#81723=CARTESIAN_POINT('Ctrl Pts',(1.17550923357461,1.37909274122413,0.599867896187775));
#81724=CARTESIAN_POINT('Ctrl Pts',(1.25478145719781,0.246049762846643,1.48363956282768));
#81725=CARTESIAN_POINT('Ctrl Pts',(1.33405368082102,-1.11162183969917,1.01293122071293));
#81726=CARTESIAN_POINT('Ctrl Pts',(1.41332590444422,-1.45444173562663,-0.382533370425969));
#81727=CARTESIAN_POINT('Ctrl Pts',(1.49259812806742,-0.4694316657159,-1.42876343278274));
#81728=CARTESIAN_POINT('Ctrl Pts',(1.57187035169063,0.944144737324904,-1.17060782271074));
#81729=CARTESIAN_POINT('Ctrl Pts',(1.65114257531383,1.49576640440171,0.156252074510604));
#81730=CARTESIAN_POINT('Ctrl Pts',(1.73041479893703,0.681831304756392,1.34046175937651));
#81731=CARTESIAN_POINT('Ctrl Pts',(1.80968702256024,-0.75458016190203,1.30089991035207));
#81732=CARTESIAN_POINT('Ctrl Pts',(1.88895924618344,-1.50209933027067,0.0736842539900608));
#81733=CARTESIAN_POINT('Ctrl Pts',(1.96823146980664,-0.878280170447616,
-1.22080124876549));
#81734=CARTESIAN_POINT('Ctrl Pts',(2.04750369342985,0.547362960556334,-1.40075892370926));
#81735=CARTESIAN_POINT('Ctrl Pts',(2.12677591705305,1.47329226116953,-0.301896770381618));
#81736=CARTESIAN_POINT('Ctrl Pts',(2.20604814067625,1.05418260801354,1.07258137045515));
#81737=CARTESIAN_POINT('Ctrl Pts',(2.28532036429946,-0.327340795261818,
1.46784869834989));
#81738=CARTESIAN_POINT('Ctrl Pts',(2.36459258792266,-1.41001907413036,0.523046715968235));
#81739=CARTESIAN_POINT('Ctrl Pts',(2.44386481154586,-1.20542361240639,-0.899269571362686));
#81740=CARTESIAN_POINT('Ctrl Pts',(2.52313703516907,0.099660923780427,-1.50059976672033));
#81741=CARTESIAN_POINT('Ctrl Pts',(2.60240925879226,1.31375984147476,-0.731960459698575));
#81742=CARTESIAN_POINT('Ctrl Pts',(2.68168148241547,1.32846531853331,0.704920165179175));
#81743=CARTESIAN_POINT('Ctrl Pts',(2.76095370603867,0.130349839849914,1.49824620528212));
#81744=CARTESIAN_POINT('Ctrl Pts',(2.84022592966187,-1.18676551918244,0.92375020468958));
#81745=CARTESIAN_POINT('Ctrl Pts',(2.91949815328508,-1.42043105915431,-0.494078827681982));
#81746=CARTESIAN_POINT('Ctrl Pts',(2.99877037690828,-0.357307286104204,
-1.46084482644884));
#81747=CARTESIAN_POINT('Ctrl Pts',(3.07804260053149,1.03200062038214,-1.09392589710831));
#81748=CARTESIAN_POINT('Ctrl Pts',(3.15731482415468,1.47918154437085,0.271671613099952));
#81749=CARTESIAN_POINT('Ctrl Pts',(3.23658704777789,0.575878860306533,1.38928268939053));
#81750=CARTESIAN_POINT('Ctrl Pts',(3.31585927140109,-0.853041679156686,
1.23848343636798));
#81751=CARTESIAN_POINT('Ctrl Pts',(3.3951314950243,-1.50342619091827,-0.0428576621857739));
#81752=CARTESIAN_POINT('Ctrl Pts',(3.47440371864751,-0.78079157970072,-1.28531750091348));
#81753=CARTESIAN_POINT('Ctrl Pts',(3.5536759422707,0.653769614982104,-1.35388071620606));
#81754=CARTESIAN_POINT('Ctrl Pts',(3.63294816589391,1.49319327315646,-0.187325998340491));
#81755=CARTESIAN_POINT('Ctrl Pts',(3.71222038951711,0.966000380289331,1.15207357520732));
#81756=CARTESIAN_POINT('Ctrl Pts',(3.76506853859925,0.0316793257180091,
1.34097184439293));
#81757=CARTESIAN_POINT('Ctrl Pts',(3.79149261314031,-0.372522267107456,
1.21727406959531));
#81758=CARTESIAN_POINT('Ctrl Pts',(0.358507386859688,-0.592743564846278,
1.2331922513677));
#81759=CARTESIAN_POINT('Ctrl Pts',(0.384931461400756,-1.00223086496478,
1.03636895657134));
#81760=CARTESIAN_POINT('Ctrl Pts',(0.437779610482891,-1.60274972266108,
0.206262289549554));
#81761=CARTESIAN_POINT('Ctrl Pts',(0.517051834106095,-1.04320983072386,
-1.23612964587239));
#81762=CARTESIAN_POINT('Ctrl Pts',(0.596324057729297,0.470088887771348,
-1.54607282736681));
#81763=CARTESIAN_POINT('Ctrl Pts',(0.675596281352501,1.55352120764973,-0.446500233285617));
#81764=CARTESIAN_POINT('Ctrl Pts',(0.754868504975704,1.21903550484369,1.06172666057649));
#81765=CARTESIAN_POINT('Ctrl Pts',(0.834140728598906,-0.228557969495404,
1.60011640659336));
#81766=CARTESIAN_POINT('Ctrl Pts',(0.913412952222111,-1.46738912067818,
0.677964854084563));
#81767=CARTESIAN_POINT('Ctrl Pts',(0.992685175845312,-1.36662352799918,
-0.863281108711857));
#81768=CARTESIAN_POINT('Ctrl Pts',(1.07195739946852,-0.0181741303108103,
-1.61631877643916));
#81769=CARTESIAN_POINT('Ctrl Pts',(1.15122962309172,1.34685268193457,-0.893782541300675));
#81770=CARTESIAN_POINT('Ctrl Pts',(1.23050184671492,1.48228094515312,0.64475196304707));
#81771=CARTESIAN_POINT('Ctrl Pts',(1.30977407033813,0.264460006296089,1.59465029995206));
#81772=CARTESIAN_POINT('Ctrl Pts',(1.38904629396133,-1.19479700091782,1.08872202886133));
#81773=CARTESIAN_POINT('Ctrl Pts',(1.46831851758453,-1.56326779636382,-0.411155761261059));
#81774=CARTESIAN_POINT('Ctrl Pts',(1.54759074120773,-0.504556069611769,
-1.53566815939119));
#81775=CARTESIAN_POINT('Ctrl Pts',(1.62686296483094,1.01478871708154,-1.25819650701018));
#81776=CARTESIAN_POINT('Ctrl Pts',(1.70613518845414,1.6076845112511,0.16794336288227));
#81777=CARTESIAN_POINT('Ctrl Pts',(1.78540741207735,0.732848140402935,1.44075946760951));
#81778=CARTESIAN_POINT('Ctrl Pts',(1.86467963570055,-0.811040303631148,
1.39823747237959));
#81779=CARTESIAN_POINT('Ctrl Pts',(1.94395185932375,-1.61449128722926,0.0791975495066015));
#81780=CARTESIAN_POINT('Ctrl Pts',(2.02322408294695,-0.943995949108369,
-1.31214556843942));
#81781=CARTESIAN_POINT('Ctrl Pts',(2.10249630657016,0.58831843737722,-1.50556826187368));
#81782=CARTESIAN_POINT('Ctrl Pts',(2.18176853019336,1.58352877953276,-0.32448566855825));
#81783=CARTESIAN_POINT('Ctrl Pts',(2.26104075381656,1.13305997911589,1.1528353967991));
#81784=CARTESIAN_POINT('Ctrl Pts',(2.34031297743977,-0.351833498128028,
1.57767791163962));
#81785=CARTESIAN_POINT('Ctrl Pts',(2.41958520106297,-1.51552128686477,0.56218277228872));
#81786=CARTESIAN_POINT('Ctrl Pts',(2.49885742468617,-1.2956173273174,-0.966555845260797));
#81787=CARTESIAN_POINT('Ctrl Pts',(2.57812964830937,0.107117878210971,-1.61287952145726));
#81788=CARTESIAN_POINT('Ctrl Pts',(2.65740187193258,1.41205962537143,-0.786728121745937));
#81789=CARTESIAN_POINT('Ctrl Pts',(2.73667409555578,1.42786541404808,0.75766458445122));
#81790=CARTESIAN_POINT('Ctrl Pts',(2.81594631917899,0.140103038786054,1.61034985889808));
#81791=CARTESIAN_POINT('Ctrl Pts',(2.89521854280218,-1.27556317487932,0.992868199188152));
#81792=CARTESIAN_POINT('Ctrl Pts',(2.9744907664254,-1.52671233046967,-0.531047412392669));
#81793=CARTESIAN_POINT('Ctrl Pts',(3.05376299004859,-0.384042179271076,
-1.57014998726522));
#81794=CARTESIAN_POINT('Ctrl Pts',(3.1330352136718,1.10921826303053,-1.17577699035228));
#81795=CARTESIAN_POINT('Ctrl Pts',(3.212307437295,1.58985871805611,0.291998966711711));
#81796=CARTESIAN_POINT('Ctrl Pts',(3.2915796609182,0.61896798948501,1.49323333838066));
#81797=CARTESIAN_POINT('Ctrl Pts',(3.37085188454141,-0.91686903181943,1.33115079482364));
#81798=CARTESIAN_POINT('Ctrl Pts',(3.45012410816461,-1.61591742790568,-0.0460644118504966));
#81799=CARTESIAN_POINT('Ctrl Pts',(3.52939633178781,-0.83921294495327,-1.38148913639031));
#81800=CARTESIAN_POINT('Ctrl Pts',(3.60866855541102,0.702686783738618,-1.45518247442965));
#81801=CARTESIAN_POINT('Ctrl Pts',(3.68794077903422,1.60491884995784,-0.201342338750495));
#81802=CARTESIAN_POINT('Ctrl Pts',(3.76721300265742,1.03827967033062,1.23827546683221));
#81803=CARTESIAN_POINT('Ctrl Pts',(3.82006115173956,0.0340496758944771,
1.44130771884574));
#81804=CARTESIAN_POINT('Ctrl Pts',(3.84648522628063,-0.400395594634544,
1.30835447425277));
#81805=CARTESIAN_POINT('Ctrl Pts',(0.4135,-0.634007094575206,1.31904027763685));
#81806=CARTESIAN_POINT('Ctrl Pts',(0.439924074541068,-1.07200063648891,
1.10851523328497));
#81807=CARTESIAN_POINT('Ctrl Pts',(0.492772223623203,-1.71432429681307,
0.220621129731974));
#81808=CARTESIAN_POINT('Ctrl Pts',(0.572044447246407,-1.11583233127307,
-1.32218215730623));
#81809=CARTESIAN_POINT('Ctrl Pts',(0.651316670869609,0.502813877035165,
-1.65370186943273));
#81810=CARTESIAN_POINT('Ctrl Pts',(0.730588894492813,1.66166876476914,-0.477583110844877));
#81811=CARTESIAN_POINT('Ctrl Pts',(0.809861118116016,1.30389801669194,1.13563820044122));
#81812=CARTESIAN_POINT('Ctrl Pts',(0.889133341739219,-0.244468911643721,
1.71150766384022));
#81813=CARTESIAN_POINT('Ctrl Pts',(0.968405565362422,-1.56954063812352,
0.725161018785134));
#81814=CARTESIAN_POINT('Ctrl Pts',(1.04767778898562,-1.46176030201119,-0.923377966453352));
#81815=CARTESIAN_POINT('Ctrl Pts',(1.12695001260883,-0.0194393127790041,
-1.72883795309242));
#81816=CARTESIAN_POINT('Ctrl Pts',(1.20622223623203,1.44061311895578,-0.956002740137796));
#81817=CARTESIAN_POINT('Ctrl Pts',(1.28549445985524,1.5854691490821,0.689636029906365));
#81818=CARTESIAN_POINT('Ctrl Pts',(1.36476668347844,0.282870249745534,1.70566103707644));
#81819=CARTESIAN_POINT('Ctrl Pts',(1.44403890710164,-1.27797216213648,1.16451283700972));
#81820=CARTESIAN_POINT('Ctrl Pts',(1.52331113072484,-1.672093857101,-0.439778152096151));
#81821=CARTESIAN_POINT('Ctrl Pts',(1.60258335434805,-0.53968047350764,-1.64257288599964));
#81822=CARTESIAN_POINT('Ctrl Pts',(1.68185557797125,1.08543269683817,-1.34578519130964));
#81823=CARTESIAN_POINT('Ctrl Pts',(1.76112780159445,1.71960261810048,0.179634651253938));
#81824=CARTESIAN_POINT('Ctrl Pts',(1.84040002521766,0.783864976049478,1.54105717584251));
#81825=CARTESIAN_POINT('Ctrl Pts',(1.91967224884086,-0.867500445360263,
1.49557503440711));
#81826=CARTESIAN_POINT('Ctrl Pts',(1.99894447246407,-1.72688324418785,0.0847108450231425));
#81827=CARTESIAN_POINT('Ctrl Pts',(2.07821669608726,-1.00971172776912,-1.40348988811335));
#81828=CARTESIAN_POINT('Ctrl Pts',(2.15748891971047,0.629273914198106,-1.6103776000381));
#81829=CARTESIAN_POINT('Ctrl Pts',(2.23676114333367,1.693765297896,-0.347074566734881));
#81830=CARTESIAN_POINT('Ctrl Pts',(2.31603336695688,1.21193735021824,1.23308942314305));
#81831=CARTESIAN_POINT('Ctrl Pts',(2.39530559058007,-0.376326200994238,
1.68750712492935));
#81832=CARTESIAN_POINT('Ctrl Pts',(2.47457781420328,-1.62102349959919,0.601318828609204));
#81833=CARTESIAN_POINT('Ctrl Pts',(2.55385003782648,-1.3858110422284,-1.03384211915891));
#81834=CARTESIAN_POINT('Ctrl Pts',(2.63312226144969,0.114574832641515,-1.72515927619419));
#81835=CARTESIAN_POINT('Ctrl Pts',(2.71239448507289,1.51035940926811,-0.8414957837933));
#81836=CARTESIAN_POINT('Ctrl Pts',(2.79166670869609,1.52726550956285,0.810409003723266));
#81837=CARTESIAN_POINT('Ctrl Pts',(2.8709389323193,0.149856237722195,1.72245351251404));
#81838=CARTESIAN_POINT('Ctrl Pts',(2.9502111559425,-1.3643608305762,1.06198619368673));
#81839=CARTESIAN_POINT('Ctrl Pts',(3.0294833795657,-1.63299360178502,-0.568015997103359));
#81840=CARTESIAN_POINT('Ctrl Pts',(3.10875560318891,-0.410777072437948,
-1.6794551480816));
#81841=CARTESIAN_POINT('Ctrl Pts',(3.1880278268121,1.18643590567891,-1.25762808359624));
#81842=CARTESIAN_POINT('Ctrl Pts',(3.26730005043532,1.70053589174136,0.312326320323468));
#81843=CARTESIAN_POINT('Ctrl Pts',(3.34657227405851,0.662057118663487,1.5971839873708));
#81844=CARTESIAN_POINT('Ctrl Pts',(3.42584449768172,-0.980696384482174,
1.42381815327929));
#81845=CARTESIAN_POINT('Ctrl Pts',(3.50511672130492,-1.72840866489308,-0.0492711615152196));
#81846=CARTESIAN_POINT('Ctrl Pts',(3.58438894492813,-0.89763431020582,-1.47766077186714));
#81847=CARTESIAN_POINT('Ctrl Pts',(3.66366116855132,0.751603952495131,-1.55648423265323));
#81848=CARTESIAN_POINT('Ctrl Pts',(3.74293339217453,1.71664442675922,-0.215358679160498));
#81849=CARTESIAN_POINT('Ctrl Pts',(3.82220561579773,1.11055896037191,1.32447735845711));
#81850=CARTESIAN_POINT('Ctrl Pts',(3.87505376487987,0.0364200260709443,
1.54164359329855));
#81851=CARTESIAN_POINT('Ctrl Pts',(3.90147783942094,-0.428268922161632,
1.39943487891024));
#81852=CARTESIAN_POINT('Ctrl Pts',(3.50284495415709,-1.4658722466537,-0.00023313482661453));
#81853=CARTESIAN_POINT('Ctrl Pts',(3.50360220987304,-1.46590495726483,-0.0140984294436677));
#81854=CARTESIAN_POINT('Ctrl Pts',(3.50435946558898,-1.46572428836199,-0.0279628793168609));
#81855=CARTESIAN_POINT('Ctrl Pts',(3.50511672130492,-1.46532755904339,-0.0418212107747877));
#81856=CARTESIAN_POINT('Ctrl Pts',(3.53154079584599,-1.45148387999733,-0.525401031632525));
#81857=CARTESIAN_POINT('Ctrl Pts',(3.55796487038706,-1.17455909510157,-1.00153090174984));
#81858=CARTESIAN_POINT('Ctrl Pts',(3.58438894492813,-0.761223658870205,
-1.25273308027284));
#81859=CARTESIAN_POINT('Ctrl Pts',(3.61081301946919,-0.347888222638836,
-1.50393525879584));
#81860=CARTESIAN_POINT('Ctrl Pts',(3.63723709401026,0.201857864928146,-1.53020974572454));
#81861=CARTESIAN_POINT('Ctrl Pts',(3.66366116855133,0.637570987755653,-1.31982606360676));
#81862=CARTESIAN_POINT('Ctrl Pts',(3.68794077903422,1.0379235105316,-1.12651621482333));
#81863=CARTESIAN_POINT('Ctrl Pts',(3.71222038951711,1.3420008677259,-0.73340182300052));
#81864=CARTESIAN_POINT('Ctrl Pts',(3.7365,1.43512958320548,-0.29838030867994));
#81865=CARTESIAN_POINT('',(0.4135,-0.684664424539457,-0.958295198918399));
#81866=CARTESIAN_POINT('Ctrl Pts',(0.4135,-0.686138785896735,-0.95953609754738));
#81867=CARTESIAN_POINT('Ctrl Pts',(0.4135,-0.714291760736759,-0.944234963869998));
#81868=CARTESIAN_POINT('Ctrl Pts',(0.4135,-0.741719807224122,-0.927747538280581));
#81869=CARTESIAN_POINT('Ctrl Pts',(0.4135,-0.768338120235236,-0.910091316634728));
#81870=CARTESIAN_POINT('Ctrl Pts',(0.4135,-0.808566078090619,-0.883407666924919));
#81871=CARTESIAN_POINT('Ctrl Pts',(0.4135,-0.846946021796831,-0.854057054820037));
#81872=CARTESIAN_POINT('Ctrl Pts',(0.4135,-0.883406381928383,-0.822336436728148));
#81873=CARTESIAN_POINT('Ctrl Pts',(0.4135,-0.900931220434468,-0.807089776866099));
#81874=CARTESIAN_POINT('Ctrl Pts',(0.4135,-0.918012314882335,-0.791294839075063));
#81875=CARTESIAN_POINT('Ctrl Pts',(0.4135,-0.934639962853447,-0.774980866858151));
#81876=CARTESIAN_POINT('Ctrl Pts',(0.4135,-0.941832779854533,-0.767923740262681));
#81877=CARTESIAN_POINT('Ctrl Pts',(0.4135,-0.948939652538661,-0.760770400163592));
#81878=CARTESIAN_POINT('Ctrl Pts',(0.4135,-0.955953136700092,-0.75353039471608));
#81879=CARTESIAN_POINT('Ctrl Pts',(0.4135,-0.991151160285013,-0.717195546496428));
#81880=CARTESIAN_POINT('Ctrl Pts',(0.4135,-1.02404693575632,-0.67863524199184));
#81881=CARTESIAN_POINT('Ctrl Pts',(0.4135,-1.05456130615998,-0.638174593980841));
#81882=CARTESIAN_POINT('Ctrl Pts',(0.4135,-1.07623986056963,-0.609429830521755));
#81883=CARTESIAN_POINT('Ctrl Pts',(0.4135,-1.09671609730046,-0.57972473829133));
#81884=CARTESIAN_POINT('Ctrl Pts',(0.4135,-1.11595336287888,-0.549162386019891));
#81885=CARTESIAN_POINT('Ctrl Pts',(0.4135,-1.12342713252684,-0.537288766048001));
#81886=CARTESIAN_POINT('Ctrl Pts',(0.4135,-1.13071381256276,-0.525285650206696));
#81887=CARTESIAN_POINT('Ctrl Pts',(0.4135,-1.13781091071671,-0.51315871424196));
#81888=CARTESIAN_POINT('Ctrl Pts',(0.4135,-1.14293138389033,-0.504409272013786));
#81889=CARTESIAN_POINT('Ctrl Pts',(0.4135,-1.14795098786502,-0.495598970025009));
#81890=CARTESIAN_POINT('Ctrl Pts',(0.4135,-1.15286514594592,-0.486737318018312));
#81891=CARTESIAN_POINT('Ctrl Pts',(0.4135,-1.17834338405788,-0.440792666630386));
#81892=CARTESIAN_POINT('Ctrl Pts',(0.4135,-1.20102252315539,-0.393415091402672));
#81893=CARTESIAN_POINT('Ctrl Pts',(0.4135,-1.22081814050263,-0.344933777036805));
#81894=CARTESIAN_POINT('Ctrl Pts',(0.4135,-1.24097727802828,-0.295562167827453));
#81895=CARTESIAN_POINT('Ctrl Pts',(0.4135,-1.25814678940821,-0.245045016208608));
#81896=CARTESIAN_POINT('Ctrl Pts',(0.4135,-1.27220121508717,-0.193691330378271));
#81897=CARTESIAN_POINT('Ctrl Pts',(0.4135,-1.28026843106556,-0.164214403725913));
#81898=CARTESIAN_POINT('Ctrl Pts',(0.4135,-1.28730858055556,-0.134461223038789));
#81899=CARTESIAN_POINT('Ctrl Pts',(0.4135,-1.29329114713789,-0.104486455012093));
#81900=CARTESIAN_POINT('Ctrl Pts',(0.4135,-1.29665686867299,-0.0876230033699474));
#81901=CARTESIAN_POINT('Ctrl Pts',(0.4135,-1.29968776382401,-0.0706893780411438));
#81902=CARTESIAN_POINT('Ctrl Pts',(0.4135,-1.30237760820265,-0.0536950834617746));
#81903=CARTESIAN_POINT('Ctrl Pts',(0.4135,-1.30392796078445,-0.0439000378129977));
#81904=CARTESIAN_POINT('Ctrl Pts',(0.4135,-1.30536494097996,-0.0340844664323464));
#81905=CARTESIAN_POINT('Ctrl Pts',(0.4135,-1.30668555024684,-0.0242654228606041));
#81906=CARTESIAN_POINT('Ctrl Pts',(0.4135,-1.31399180339102,0.0300583046551521));
#81907=CARTESIAN_POINT('Ctrl Pts',(0.4135,-1.3177582625026,0.0845978055922513));
#81908=CARTESIAN_POINT('Ctrl Pts',(0.4135,-1.31787095116813,0.139023202239183));
#81909=CARTESIAN_POINT('Ctrl Pts',(0.4135,-1.31789100087815,0.148706637709421));
#81910=CARTESIAN_POINT('Ctrl Pts',(0.4135,-1.317795273435,0.158386530765053));
#81911=CARTESIAN_POINT('Ctrl Pts',(0.4135,-1.31758297383669,0.16806110450681));
#81912=CARTESIAN_POINT('Ctrl Pts',(0.4135,-1.31643127886986,0.220544283812512));
#81913=CARTESIAN_POINT('Ctrl Pts',(0.4135,-1.31185321745701,0.272870263476887));
#81914=CARTESIAN_POINT('Ctrl Pts',(0.4135,-1.30405110481389,0.324821294688041));
#81915=CARTESIAN_POINT('Ctrl Pts',(0.4135,-1.30004755732558,0.351479256452338));
#81916=CARTESIAN_POINT('Ctrl Pts',(0.4135,-1.29519424013352,0.378038631051489));
#81917=CARTESIAN_POINT('Ctrl Pts',(0.4135,-1.28951334705064,0.404470290630908));
#81918=CARTESIAN_POINT('Ctrl Pts',(0.4135,-1.28605512944955,0.420560442135318));
#81919=CARTESIAN_POINT('Ctrl Pts',(0.4135,-1.28229017007228,0.436603265746692));
#81920=CARTESIAN_POINT('Ctrl Pts',(0.4135,-1.27822287787089,0.452592132714455));
#81921=CARTESIAN_POINT('Ctrl Pts',(0.4135,-1.27553847269057,0.463144754751541));
#81922=CARTESIAN_POINT('Ctrl Pts',(0.4135,-1.27272184329057,0.473675296709342));
#81923=CARTESIAN_POINT('Ctrl Pts',(0.4135,-1.26977956742198,0.48416381510515));
#81924=CARTESIAN_POINT('Ctrl Pts',(0.4135,-1.25497166843981,0.536950476796429));
#81925=CARTESIAN_POINT('Ctrl Pts',(0.4135,-1.23696085773443,0.588774472230241));
#81926=CARTESIAN_POINT('Ctrl Pts',(0.4135,-1.21598695973147,0.639400292991206));
#81927=CARTESIAN_POINT('Ctrl Pts',(0.4135,-1.19455580907984,0.691129808956144));
#81928=CARTESIAN_POINT('Ctrl Pts',(0.4135,-1.17003074758714,0.741609292791885));
#81929=CARTESIAN_POINT('Ctrl Pts',(0.4135,-1.1426126898322,0.790587857943637));
#81930=CARTESIAN_POINT('Ctrl Pts',(0.4135,-1.12720475153753,0.818112007041462));
#81931=CARTESIAN_POINT('Ctrl Pts',(0.4135,-1.11088223265367,0.845162088565469));
#81932=CARTESIAN_POINT('Ctrl Pts',(0.4135,-1.09367386201465,0.871691839113621));
#81933=CARTESIAN_POINT('Ctrl Pts',(0.4135,-1.08240277099321,0.889068221775127));
#81934=CARTESIAN_POINT('Ctrl Pts',(0.4135,-1.07075155454919,0.90622135373255));
#81935=CARTESIAN_POINT('Ctrl Pts',(0.4135,-1.05872722186107,0.923137718332686));
#81936=CARTESIAN_POINT('Ctrl Pts',(0.4135,-1.05266396799753,0.931667772821302));
#81937=CARTESIAN_POINT('Ctrl Pts',(0.4135,-1.04650431325987,0.940139649745939));
#81938=CARTESIAN_POINT('Ctrl Pts',(0.4135,-1.04025403002402,0.948544932930425));
#81939=CARTESIAN_POINT('Ctrl Pts',(0.4135,-1.00551853942241,0.995256677669289));
#81940=CARTESIAN_POINT('Ctrl Pts',(0.4135,-0.968096092333637,1.03977033457125));
#81941=CARTESIAN_POINT('Ctrl Pts',(0.4135,-0.928214711176929,1.08182781872808));
#81942=CARTESIAN_POINT('Ctrl Pts',(0.4135,-0.888231183206945,1.12399302327614));
#81943=CARTESIAN_POINT('Ctrl Pts',(0.4135,-0.845775625163952,1.16369052758893));
#81944=CARTESIAN_POINT('Ctrl Pts',(0.4135,-0.801028754132348,1.20064269443073));
#81945=CARTESIAN_POINT('Ctrl Pts',(0.4135,-0.757313300281664,1.23674311233737));
#81946=CARTESIAN_POINT('Ctrl Pts',(0.4135,-0.711410323916766,1.27022418935027));
#81947=CARTESIAN_POINT('Ctrl Pts',(0.4135,-0.663450030477264,1.30079597351158));
#81948=CARTESIAN_POINT('Ctrl Pts',(0.4135,-0.653720195627844,1.30699815430759));
#81949=CARTESIAN_POINT('Ctrl Pts',(0.4135,-0.64390557580449,1.3130804666773));
#81950=CARTESIAN_POINT('Ctrl Pts',(0.4135,-0.634007094575209,1.31904027763685));
#81951=CARTESIAN_POINT('Ctrl Pts',(0.4135,-0.68613878589674,-0.959536097547376));
#81952=CARTESIAN_POINT('Ctrl Pts',(0.437779610482891,-0.393693948037641,
-1.16605720471058));
#81953=CARTESIAN_POINT('Ctrl Pts',(0.488483295506851,0.429867162043437,
-1.3052106562365));
#81954=CARTESIAN_POINT('Ctrl Pts',(0.565611055071876,1.33722609341091,-0.384334478167097));
#81955=CARTESIAN_POINT('Ctrl Pts',(0.644883278695081,1.0493104811472,0.913903580847046));
#81956=CARTESIAN_POINT('Ctrl Pts',(0.724155502318283,-0.196736085198769,
1.37733389209964));
#81957=CARTESIAN_POINT('Ctrl Pts',(0.78848344766531,-1.06205941565968,0.733211202865703));
#81958=CARTESIAN_POINT('Ctrl Pts',(0.826387318471269,-1.1764950713461,0.170924181182572));
#81959=CARTESIAN_POINT('Ctrl Pts',(0.837867114736159,-1.17596232425638,
0.000418044704970002));
#81960=CARTESIAN_POINT('Origin',(0.4135,-3.28582941601228E-17,0.));
#81961=CARTESIAN_POINT('',(0.4135,-1.4635,-1.79227059055215E-16));
#81962=CARTESIAN_POINT('Origin',(0.4135,0.,0.));
#81963=CARTESIAN_POINT('Origin',(0.4135,0.,0.));
#81964=CARTESIAN_POINT('',(0.4135,0.684664424539459,-0.958295198918398));
#81965=CARTESIAN_POINT('Ctrl Pts',(0.4135,0.635547413990925,1.32087379520599));
#81966=CARTESIAN_POINT('Ctrl Pts',(0.4135,0.669353330290829,1.30074697282028));
#81967=CARTESIAN_POINT('Ctrl Pts',(0.4135,0.702232179962959,1.27920433805169));
#81968=CARTESIAN_POINT('Ctrl Pts',(0.4135,0.734081619959607,1.2562406920021));
#81969=CARTESIAN_POINT('Ctrl Pts',(0.4135,0.780755752573622,1.22258834957055));
#81970=CARTESIAN_POINT('Ctrl Pts',(0.4135,0.825221151134185,1.18588514692087));
#81971=CARTESIAN_POINT('Ctrl Pts',(0.4135,0.8673274179155,1.14644100535051));
#81972=CARTESIAN_POINT('Ctrl Pts',(0.4135,0.881456789981801,1.13320494823394));
#81973=CARTESIAN_POINT('Ctrl Pts',(0.4135,0.895320162781675,1.11966001938105));
#81974=CARTESIAN_POINT('Ctrl Pts',(0.4135,0.908910741618978,1.10581733905333));
#81975=CARTESIAN_POINT('Ctrl Pts',(0.4135,0.917246814053772,1.09732663477318));
#81976=CARTESIAN_POINT('Ctrl Pts',(0.4135,0.925480243365935,1.08872390441625));
#81977=CARTESIAN_POINT('Ctrl Pts',(0.4135,0.933609350058259,1.08001167838196));
#81978=CARTESIAN_POINT('Ctrl Pts',(0.4135,0.942209207594102,1.07079493347373));
#81979=CARTESIAN_POINT('Ctrl Pts',(0.4135,0.950686065026906,1.06146229962268));
#81980=CARTESIAN_POINT('Ctrl Pts',(0.4135,0.95903640633612,1.05201957849277));
#81981=CARTESIAN_POINT('Ctrl Pts',(0.4135,0.997169509051934,1.00889795730031));
#81982=CARTESIAN_POINT('Ctrl Pts',(0.4135,1.03268280360029,0.963466516297889));
#81983=CARTESIAN_POINT('Ctrl Pts',(0.4135,1.06542315300417,0.916036856053426));
#81984=CARTESIAN_POINT('Ctrl Pts',(0.4135,1.08701635006398,0.884755638266009));
#81985=CARTESIAN_POINT('Ctrl Pts',(0.4135,1.10740246223309,0.852604627640892));
#81986=CARTESIAN_POINT('Ctrl Pts',(0.4135,1.12652571878095,0.819669470930706));
#81987=CARTESIAN_POINT('Ctrl Pts',(0.4135,1.13332764876214,0.807954801449515));
#81988=CARTESIAN_POINT('Ctrl Pts',(0.4135,1.13996971756187,0.796140912143825));
#81989=CARTESIAN_POINT('Ctrl Pts',(0.4135,1.14644910558472,0.78423162968392));
#81990=CARTESIAN_POINT('Ctrl Pts',(0.4135,1.15259842154092,0.772929028203779));
#81991=CARTESIAN_POINT('Ctrl Pts',(0.4135,1.15860189203148,0.761538847236137));
#81992=CARTESIAN_POINT('Ctrl Pts',(0.4135,1.16444748634856,0.750083887702724));
#81993=CARTESIAN_POINT('Ctrl Pts',(0.4135,1.19001813114109,0.699975945643586));
#81994=CARTESIAN_POINT('Ctrl Pts',(0.4135,1.21261752532289,0.648548155053135));
#81995=CARTESIAN_POINT('Ctrl Pts',(0.4135,1.2321019520388,0.596089578702456));
#81996=CARTESIAN_POINT('Ctrl Pts',(0.4135,1.25109784966556,0.544946285623718));
#81997=CARTESIAN_POINT('Ctrl Pts',(0.4135,1.26713314523672,0.492822207443129));
#81998=CARTESIAN_POINT('Ctrl Pts',(0.4135,1.28002636999895,0.439979726788032));
#81999=CARTESIAN_POINT('Ctrl Pts',(0.4135,1.28761762878201,0.408867188785392));
#82000=CARTESIAN_POINT('Ctrl Pts',(0.4135,1.29411873111552,0.37750558303088));
#82001=CARTESIAN_POINT('Ctrl Pts',(0.4135,1.2994842302109,0.345949663324928));
#82002=CARTESIAN_POINT('Ctrl Pts',(0.4135,1.3033411938025,0.323265840023198));
#82003=CARTESIAN_POINT('Ctrl Pts',(0.4135,1.30661121725092,0.300481627400674));
#82004=CARTESIAN_POINT('Ctrl Pts',(0.4135,1.30927531071834,0.277618009171112));
#82005=CARTESIAN_POINT('Ctrl Pts',(0.4135,1.31040225052168,0.267946456071913));
#82006=CARTESIAN_POINT('Ctrl Pts',(0.4135,1.31142057568754,0.258261278874394));
#82007=CARTESIAN_POINT('Ctrl Pts',(0.4135,1.31232784965945,0.248577394511979));
#82008=CARTESIAN_POINT('Ctrl Pts',(0.4135,1.31724670409264,0.19607548329048));
#82009=CARTESIAN_POINT('Ctrl Pts',(0.4135,1.31891803803387,0.143509146220101));
#82010=CARTESIAN_POINT('Ctrl Pts',(0.4135,1.3171831677328,0.0911229999231752));
#82011=CARTESIAN_POINT('Ctrl Pts',(0.4135,1.31683748835986,0.0806848650426602));
#82012=CARTESIAN_POINT('Ctrl Pts',(0.4135,1.31635641176535,0.0702539051829255));
#82013=CARTESIAN_POINT('Ctrl Pts',(0.4135,1.31573843466204,0.059832098621419));
#82014=CARTESIAN_POINT('Ctrl Pts',(0.4135,1.31241181507788,0.00373069029382706));
#82015=CARTESIAN_POINT('Ctrl Pts',(0.4135,1.3051227222334,-0.0521077326158235));
#82016=CARTESIAN_POINT('Ctrl Pts',(0.4135,1.29405566219162,-0.107356325259506));
#82017=CARTESIAN_POINT('Ctrl Pts',(0.4135,1.28930638402934,-0.1310655066996));
#82018=CARTESIAN_POINT('Ctrl Pts',(0.4135,1.28386065917644,-0.154665702263389));
#82019=CARTESIAN_POINT('Ctrl Pts',(0.4135,1.27773018452238,-0.178129059070878));
#82020=CARTESIAN_POINT('Ctrl Pts',(0.4135,1.27333395871588,-0.194954871185749));
#82021=CARTESIAN_POINT('Ctrl Pts',(0.413500000000001,1.26858556750922,-0.21171028751553));
#82022=CARTESIAN_POINT('Ctrl Pts',(0.413500000000001,1.26348886213856,-0.228384538292229));
#82023=CARTESIAN_POINT('Ctrl Pts',(0.413500000000001,1.26053100374918,-0.238061392055544));
#82024=CARTESIAN_POINT('Ctrl Pts',(0.4135,1.25745837360604,-0.247702450741358));
#82025=CARTESIAN_POINT('Ctrl Pts',(0.4135,1.25427370148489,-0.257301724258028));
#82026=CARTESIAN_POINT('Ctrl Pts',(0.4135,1.23773749554111,-0.30714533695771));
#82027=CARTESIAN_POINT('Ctrl Pts',(0.413500000000001,1.21817302763353,-0.35590112182507));
#82028=CARTESIAN_POINT('Ctrl Pts',(0.413500000000001,1.19575248320236,-0.403310675257065));
#82029=CARTESIAN_POINT('Ctrl Pts',(0.413500000000001,1.17344343049265,-0.45048447291861));
#82030=CARTESIAN_POINT('Ctrl Pts',(0.4135,1.14830584182414,-0.496326289088077));
#82031=CARTESIAN_POINT('Ctrl Pts',(0.4135,1.12047022689924,-0.540548779036441));
#82032=CARTESIAN_POINT('Ctrl Pts',(0.4135,1.1065437748044,-0.562673757753156));
#82033=CARTESIAN_POINT('Ctrl Pts',(0.413500000000001,1.09194143893574,-0.584392804363012));
#82034=CARTESIAN_POINT('Ctrl Pts',(0.413500000000001,1.07667679045606,-0.605665778680436));
#82035=CARTESIAN_POINT('Ctrl Pts',(0.413500000000001,1.06542302105988,-0.621349149814594));
#82036=CARTESIAN_POINT('Ctrl Pts',(0.413500000000001,1.05380922812795,-0.636790009908271));
#82037=CARTESIAN_POINT('Ctrl Pts',(0.413500000000001,1.04184035177154,-0.651971132742421));
#82038=CARTESIAN_POINT('Ctrl Pts',(0.413500000000001,1.03605335611918,-0.659311261357929));
#82039=CARTESIAN_POINT('Ctrl Pts',(0.4135,1.03018390785768,-0.666589788171434));
#82040=CARTESIAN_POINT('Ctrl Pts',(0.4135,1.02424093292914,-0.673795048425256));
#82041=CARTESIAN_POINT('Ctrl Pts',(0.4135,0.992152443281526,-0.712699119507982));
#82042=CARTESIAN_POINT('Ctrl Pts',(0.4135,0.957861254279335,-0.749549587746932));
#82043=CARTESIAN_POINT('Ctrl Pts',(0.4135,0.921497384787766,-0.78409445806545));
#82044=CARTESIAN_POINT('Ctrl Pts',(0.4135,0.885875868446326,-0.817934109339342));
#82045=CARTESIAN_POINT('Ctrl Pts',(0.4135,0.848264687334309,-0.849561915469862));
#82046=CARTESIAN_POINT('Ctrl Pts',(0.4135,0.808762330645478,-0.87869744037182));
#82047=CARTESIAN_POINT('Ctrl Pts',(0.4135,0.769259973956647,-0.907832965273778));
#82048=CARTESIAN_POINT('Ctrl Pts',(0.4135,0.727865816193214,-0.934476889771254));
#82049=CARTESIAN_POINT('Ctrl Pts',(0.4135,0.684664424539464,-0.958295198918394));
#82050=CARTESIAN_POINT('Origin',(0.4135,0.,0.));
#82051=CARTESIAN_POINT('Origin',(-0.510867114736157,0.,0.));
#82052=CARTESIAN_POINT('Ctrl Pts',(0.4135,0.68466442453946,-0.958295198918397));
#82053=CARTESIAN_POINT('Ctrl Pts',(0.439924074541068,1.00287086257571,-0.730949149362124));
#82054=CARTESIAN_POINT('Ctrl Pts',(0.492772223623204,1.38961280228995,0.0616289067023483));
#82055=CARTESIAN_POINT('Ctrl Pts',(0.572044447246405,0.702229323936485,
1.20223305857378));
#82056=CARTESIAN_POINT('Ctrl Pts',(0.65131667086961,-0.626827250790123,
1.2417271038667));
#82057=CARTESIAN_POINT('Ctrl Pts',(0.707012816875422,-1.15833492858927,
0.474239310809062));
#82058=CARTESIAN_POINT('Ctrl Pts',(0.736284888340166,-1.17941005150351,
0.0427943559881212));
#82059=CARTESIAN_POINT('Ctrl Pts',(0.739132885263843,-1.17911213255423,
0.000786107540026912));
#82060=CARTESIAN_POINT('Ctrl Pts',(0.248522160579064,0.850780204044571,
-1.1908002747757));
#82061=CARTESIAN_POINT('Ctrl Pts',(0.274946235120132,1.24619104850736,-0.90829469759412));
#82062=CARTESIAN_POINT('Ctrl Pts',(0.327794384202267,1.72676572799944,0.0765815367937832));
#82063=CARTESIAN_POINT('Ctrl Pts',(0.407066607825471,0.872606763388711,
1.49392322752938));
#82064=CARTESIAN_POINT('Ctrl Pts',(0.486338831448673,-0.778910364280483,
1.54299946211752));
#82065=CARTESIAN_POINT('Ctrl Pts',(0.565611055071877,-1.71894759058321,
0.185602144369403));
#82066=CARTESIAN_POINT('Ctrl Pts',(0.64488327869508,-1.08987267889964,-1.34238662655454));
#82067=CARTESIAN_POINT('Ctrl Pts',(0.724155502318283,0.534302828499086,
-1.6442454361086));
#82068=CARTESIAN_POINT('Ctrl Pts',(0.803427725941486,1.67063323497912,-0.445309606403874));
#82069=CARTESIAN_POINT('Ctrl Pts',(0.882699949564689,1.28179129667979,1.1603365151821));
#82070=CARTESIAN_POINT('Ctrl Pts',(0.961972173187892,-0.277274268110296,
1.70656878530735));
#82071=CARTESIAN_POINT('Ctrl Pts',(1.0412443968111,-1.58319498499271,0.694838588358626));
#82072=CARTESIAN_POINT('Ctrl Pts',(1.1205166204343,-1.44374543633381,-0.95126705305996));
#82073=CARTESIAN_POINT('Ctrl Pts',(1.1997888440575,0.0137705542152546,-1.72890285984628));
#82074=CARTESIAN_POINT('Ctrl Pts',(1.2790610676807,1.45871359983909,-0.928147203425756));
#82075=CARTESIAN_POINT('Ctrl Pts',(1.35833329130391,1.57192783763916,0.719961917183323));
#82076=CARTESIAN_POINT('Ctrl Pts',(1.43760551492711,0.250053655582714,1.71078153521168));
#82077=CARTESIAN_POINT('Ctrl Pts',(1.51687773855032,-1.30010630151546,1.13974783301697));
#82078=CARTESIAN_POINT('Ctrl Pts',(1.59614996217352,-1.6633371234547,-0.471816683068196));
#82079=CARTESIAN_POINT('Ctrl Pts',(1.67542218579672,-0.508027887927404,
-1.65263691735815));
#82080=CARTESIAN_POINT('Ctrl Pts',(1.75469440941992,1.11108428040716,-1.32468600981118));
#82081=CARTESIAN_POINT('Ctrl Pts',(1.83396663304312,1.71583448087688,0.212634185438564));
#82082=CARTESIAN_POINT('Ctrl Pts',(1.91323885666633,0.754117317251402,1.55583042366493));
#82083=CARTESIAN_POINT('Ctrl Pts',(1.99251108028953,-0.896069614137905,
1.47863467995162));
#82084=CARTESIAN_POINT('Ctrl Pts',(2.07178330391274,-1.72819173027205,0.0515226047396124));
#82085=CARTESIAN_POINT('Ctrl Pts',(2.15105552753594,-0.9825649808076,-1.42262690860033));
#82086=CARTESIAN_POINT('Ctrl Pts',(2.23032775115914,0.660092369291553,-1.59799229245964));
#82087=CARTESIAN_POINT('Ctrl Pts',(2.30959997478234,1.70011975464927,-0.314474061535004));
#82088=CARTESIAN_POINT('Ctrl Pts',(2.38887219840555,1.18802663996317,1.25614253626802));
#82089=CARTESIAN_POINT('Ctrl Pts',(2.46814442202875,-0.408673070957845,
1.67996661847221));
#82090=CARTESIAN_POINT('Ctrl Pts',(2.54741664565196,-1.63227510030183,0.570068670272428));
#82091=CARTESIAN_POINT('Ctrl Pts',(2.62668886927516,-1.36569605607521,-1.0602719327417));
#82092=CARTESIAN_POINT('Ctrl Pts',(2.70596109289836,0.147694007720903,-1.72264014746723));
#82093=CARTESIAN_POINT('Ctrl Pts',(2.78523331652156,1.52624377360986,-0.812326701804879));
#82094=CARTESIAN_POINT('Ctrl Pts',(2.86450554014477,1.51141902517799,0.839596582593152));
#82095=CARTESIAN_POINT('Ctrl Pts',(2.94377776376797,0.116735341773671,1.72501590843657));
#82096=CARTESIAN_POINT('Ctrl Pts',(3.02304998739117,-1.38449836206145,1.03557825594721));
#82097=CARTESIAN_POINT('Ctrl Pts',(3.10232221101438,-1.62180155186573,-0.599274130156542));
#82098=CARTESIAN_POINT('Ctrl Pts',(3.18159443463758,-0.378400318371864,
-1.68704749501265));
#82099=CARTESIAN_POINT('Ctrl Pts',(3.26086665826079,1.2103003861222,-1.23458314505688));
#82100=CARTESIAN_POINT('Ctrl Pts',(3.34013888188398,1.69436502395503,0.344893428412662));
#82101=CARTESIAN_POINT('Ctrl Pts',(3.41941110550719,0.630982028908847,1.60968650810039));
#82102=CARTESIAN_POINT('Ctrl Pts',(3.49868332913039,-1.00734708824837,1.4045641813303));
#82103=CARTESIAN_POINT('Ctrl Pts',(3.5779555527536,-1.72814876805798,-0.0821645222904032));
#82104=CARTESIAN_POINT('Ctrl Pts',(3.6572277763768,-0.867017569131943,-1.49528095887952));
#82105=CARTESIAN_POINT('Ctrl Pts',(3.71007592545893,0.228448785913636,-1.5250582084865));
#82106=CARTESIAN_POINT('Ctrl Pts',(3.7365,0.66187319412785,-1.30528009442227));
#82107=CARTESIAN_POINT('Ctrl Pts',(0.303514773719376,0.795408277542867,
-1.11329858282326));
#82108=CARTESIAN_POINT('Ctrl Pts',(0.329938848260444,1.16508431986348,-0.849179514850122));
#82109=CARTESIAN_POINT('Ctrl Pts',(0.382786997342579,1.61438141942961,0.0715973267633055));
#82110=CARTESIAN_POINT('Ctrl Pts',(0.462059220965783,0.815814283571302,
1.39669317121085));
#82111=CARTESIAN_POINT('Ctrl Pts',(0.541331444588985,-0.72821599311703,
1.44257534270058));
#82112=CARTESIAN_POINT('Ctrl Pts',(0.620603668212189,-1.60707211535051,
0.173522469445461));
#82113=CARTESIAN_POINT('Ctrl Pts',(0.699875891835391,-1.01893972866719,
-1.25501913343577));
#82114=CARTESIAN_POINT('Ctrl Pts',(0.779148115458596,0.49952842165622,-1.53723185374485));
#82115=CARTESIAN_POINT('Ctrl Pts',(0.858420339081797,1.56190223693897,-0.416327208036965));
#82116=CARTESIAN_POINT('Ctrl Pts',(0.937692562705002,1.19836757204108,1.08481751752505));
#82117=CARTESIAN_POINT('Ctrl Pts',(1.0169647863282,-0.259228231870117,1.5954989685663));
#82118=CARTESIAN_POINT('Ctrl Pts',(1.09623700995141,-1.48015479208491,0.649615919727836));
#82119=CARTESIAN_POINT('Ctrl Pts',(1.17550923357461,-1.34978113649726,-0.88935507027625));
#82120=CARTESIAN_POINT('Ctrl Pts',(1.25478145719781,0.0128743155483621,
-1.6163794588211));
#82121=CARTESIAN_POINT('Ctrl Pts',(1.33405368082102,1.36377511648776,-0.867739946079459));
#82122=CARTESIAN_POINT('Ctrl Pts',(1.41332590444422,1.46962095240846,0.673104129269616));
#82123=CARTESIAN_POINT('Ctrl Pts',(1.49259812806742,0.233779237616018,1.59943753710515));
#82124=CARTESIAN_POINT('Ctrl Pts',(1.57187035169063,-1.21549056853332,1.06556882304439));
#82125=CARTESIAN_POINT('Ctrl Pts',(1.65114257531383,-1.55508098337335,-0.441109105984328));
#82126=CARTESIAN_POINT('Ctrl Pts',(1.73041479893703,-0.474963551524882,
-1.54507718631724));
#82127=CARTESIAN_POINT('Ctrl Pts',(1.80968702256023,1.03877080059248,-1.23847053838343));
#82128=CARTESIAN_POINT('Ctrl Pts',(1.88895924618344,1.60416161835313,0.198795165170016));
#82129=CARTESIAN_POINT('Ctrl Pts',(1.96823146980664,0.705036569408422,1.45457121775165));
#82130=CARTESIAN_POINT('Ctrl Pts',(2.04750369342984,-0.837750085100231,
1.38239965892983));
#82131=CARTESIAN_POINT('Ctrl Pts',(2.12677591705305,-1.61571461219319,0.0481693228117334));
#82132=CARTESIAN_POINT('Ctrl Pts',(2.20604814067625,-0.918616012975739,
-1.3300370807601));
#82133=CARTESIAN_POINT('Ctrl Pts',(2.28532036429946,0.617131113278558,-1.4939890359808));
#82134=CARTESIAN_POINT('Ctrl Pts',(2.36459258792266,1.58946966470712,-0.294006924971143));
#82135=CARTESIAN_POINT('Ctrl Pts',(2.44386481154586,1.11070546643635,1.17438812794583));
#82136=CARTESIAN_POINT('Ctrl Pts',(2.52313703516906,-0.382075113999367,
1.5706281692686));
#82137=CARTESIAN_POINT('Ctrl Pts',(2.60240925879227,-1.52604059172393,0.53296648998992));
#82138=CARTESIAN_POINT('Ctrl Pts',(2.68168148241547,-1.27681149895791,-0.991265508694116));
#82139=CARTESIAN_POINT('Ctrl Pts',(2.76095370603867,0.138081534720963,-1.61052434695731));
#82140=CARTESIAN_POINT('Ctrl Pts',(2.84022592966188,1.42691017645486,-0.75945747163958));
#82141=CARTESIAN_POINT('Ctrl Pts',(2.91949815328508,1.41305027755367,0.784952527593498));
#82142=CARTESIAN_POINT('Ctrl Pts',(2.99877037690829,0.109137773407462,1.61274548460426));
#82143=CARTESIAN_POINT('Ctrl Pts',(3.07804260053148,-1.29439008123716,0.968178987837214));
#82144=CARTESIAN_POINT('Ctrl Pts',(3.15731482415469,-1.51624870060833,-0.5602711503838));
#82145=CARTESIAN_POINT('Ctrl Pts',(3.23658704777789,-0.353772624265322,
-1.57724819614011));
#82146=CARTESIAN_POINT('Ctrl Pts',(3.3158592714011,1.13152955470564,-1.15423190175885));
#82147=CARTESIAN_POINT('Ctrl Pts',(3.3951314950243,1.58408947319882,0.322446486795784));
#82148=CARTESIAN_POINT('Ctrl Pts',(3.4744037186475,0.589915381656662,1.5049221487587));
#82149=CARTESIAN_POINT('Ctrl Pts',(3.55367594227071,-0.941785209084957,
1.31314994267521));
#82150=CARTESIAN_POINT('Ctrl Pts',(3.6329481658939,-1.61567444611912,-0.0768169508874945));
#82151=CARTESIAN_POINT('Ctrl Pts',(3.71222038951711,-0.810588854776071,
-1.39796253637643));
#82152=CARTESIAN_POINT('Ctrl Pts',(3.76506853859925,0.213580492877578,-1.42580177230041));
#82153=CARTESIAN_POINT('Ctrl Pts',(3.79149261314031,0.618796035439312,-1.22032763183687));
#82154=CARTESIAN_POINT('Ctrl Pts',(0.358507386859688,0.740036351041164,
-1.03579689087083));
#82155=CARTESIAN_POINT('Ctrl Pts',(0.384931461400756,1.08397759121959,-0.790064332106122));
#82156=CARTESIAN_POINT('Ctrl Pts',(0.437779610482892,1.50199711085978,0.0666131167328262));
#82157=CARTESIAN_POINT('Ctrl Pts',(0.517051834106093,0.759021803753894,
1.29946311489232));
#82158=CARTESIAN_POINT('Ctrl Pts',(0.596324057729298,-0.677521621953577,
1.34215122328364));
#82159=CARTESIAN_POINT('Ctrl Pts',(0.675596281352501,-1.49519664011782,
0.16144279452152));
#82160=CARTESIAN_POINT('Ctrl Pts',(0.754868504975703,-0.94800677843474,
-1.167651640317));
#82161=CARTESIAN_POINT('Ctrl Pts',(0.834140728598908,0.464754014813354,
-1.4302182713811));
#82162=CARTESIAN_POINT('Ctrl Pts',(0.913412952222109,1.45317123889882,-0.387344809670057));
#82163=CARTESIAN_POINT('Ctrl Pts',(0.992685175845314,1.11494384740237,1.009298519868));
#82164=CARTESIAN_POINT('Ctrl Pts',(1.07195739946851,-0.241182195629937,
1.48442915182525));
#82165=CARTESIAN_POINT('Ctrl Pts',(1.15122962309172,-1.37711459917712,0.604393251097046));
#82166=CARTESIAN_POINT('Ctrl Pts',(1.23050184671492,-1.25581683666071,-0.827443087492541));
#82167=CARTESIAN_POINT('Ctrl Pts',(1.30977407033813,0.0119780768814665,
-1.50385605779591));
#82168=CARTESIAN_POINT('Ctrl Pts',(1.38904629396133,1.26883663313643,-0.807332688733162));
#82169=CARTESIAN_POINT('Ctrl Pts',(1.46831851758453,1.36731406717776,0.62624634135591));
#82170=CARTESIAN_POINT('Ctrl Pts',(1.54759074120774,0.217504819649325,1.48809353899862));
#82171=CARTESIAN_POINT('Ctrl Pts',(1.62686296483094,-1.1308748355512,0.991389813071809));
#82172=CARTESIAN_POINT('Ctrl Pts',(1.70613518845414,-1.44682484329199,-0.410401528900456));
#82173=CARTESIAN_POINT('Ctrl Pts',(1.78540741207734,-0.441899215122363,
-1.43751745527634));
#82174=CARTESIAN_POINT('Ctrl Pts',(1.86467963570055,0.966457320777803,-1.15225506695567));
#82175=CARTESIAN_POINT('Ctrl Pts',(1.94395185932375,1.49248875582936,0.184956144901466));
#82176=CARTESIAN_POINT('Ctrl Pts',(2.02322408294696,0.655955821565445,1.35331201183838));
#82177=CARTESIAN_POINT('Ctrl Pts',(2.10249630657015,-0.77943055606256,1.28616463790804));
#82178=CARTESIAN_POINT('Ctrl Pts',(2.18176853019336,-1.50323749411433,0.044816040883855));
#82179=CARTESIAN_POINT('Ctrl Pts',(2.26104075381656,-0.854667045143881,
-1.23744725291987));
#82180=CARTESIAN_POINT('Ctrl Pts',(2.34031297743977,0.574169857265563,-1.38998577950196));
#82181=CARTESIAN_POINT('Ctrl Pts',(2.41958520106297,1.47881957476497,-0.273539788407282));
#82182=CARTESIAN_POINT('Ctrl Pts',(2.49885742468617,1.03338429290954,1.09263371962364));
#82183=CARTESIAN_POINT('Ctrl Pts',(2.57812964830938,-0.35547715704089,1.46128972006499));
#82184=CARTESIAN_POINT('Ctrl Pts',(2.65740187193258,-1.41980608314604,0.495864309707411));
#82185=CARTESIAN_POINT('Ctrl Pts',(2.73667409555578,-1.18792694184062,-0.922259084646528));
#82186=CARTESIAN_POINT('Ctrl Pts',(2.81594631917899,0.128469061721023,-1.4984085464474));
#82187=CARTESIAN_POINT('Ctrl Pts',(2.89521854280219,1.32757657929986,-0.706588241474279));
#82188=CARTESIAN_POINT('Ctrl Pts',(2.97449076642539,1.31468152992934,0.730308472593842));
#82189=CARTESIAN_POINT('Ctrl Pts',(3.05376299004859,0.101540205041254,1.50047506077196));
#82190=CARTESIAN_POINT('Ctrl Pts',(3.1330352136718,-1.20428180041287,0.900779719727221));
#82191=CARTESIAN_POINT('Ctrl Pts',(3.212307437295,-1.41069584935093,-0.521268170611058));
#82192=CARTESIAN_POINT('Ctrl Pts',(3.2915796609182,-0.32914493015878,-1.46744889726758));
#82193=CARTESIAN_POINT('Ctrl Pts',(3.37085188454141,1.05275872328908,-1.07388065846081));
#82194=CARTESIAN_POINT('Ctrl Pts',(3.45012410816461,1.4738139224426,0.299999545178905));
#82195=CARTESIAN_POINT('Ctrl Pts',(3.52939633178781,0.548848734404479,1.40015778941701));
#82196=CARTESIAN_POINT('Ctrl Pts',(3.60866855541102,-0.876223329921544,
1.22173570402013));
#82197=CARTESIAN_POINT('Ctrl Pts',(3.68794077903421,-1.50320012418026,-0.0714693794845846));
#82198=CARTESIAN_POINT('Ctrl Pts',(3.76721300265743,-0.754160140420199,
-1.30064411387334));
#82199=CARTESIAN_POINT('Ctrl Pts',(3.82006115173956,0.198712199841519,-1.32654533611433));
#82200=CARTESIAN_POINT('Ctrl Pts',(3.84648522628063,0.575718876750774,-1.13537516925148));
#82201=CARTESIAN_POINT('Ctrl Pts',(0.4135,0.68466442453946,-0.958295198918397));
#82202=CARTESIAN_POINT('Ctrl Pts',(0.439924074541068,1.00287086257571,-0.730949149362124));
#82203=CARTESIAN_POINT('Ctrl Pts',(0.492772223623204,1.38961280228995,0.0616289067023483));
#82204=CARTESIAN_POINT('Ctrl Pts',(0.572044447246405,0.702229323936485,
1.20223305857378));
#82205=CARTESIAN_POINT('Ctrl Pts',(0.65131667086961,-0.626827250790123,
1.2417271038667));
#82206=CARTESIAN_POINT('Ctrl Pts',(0.730588894492812,-1.38332116488512,
0.149363119597578));
#82207=CARTESIAN_POINT('Ctrl Pts',(0.809861118116015,-0.877073828202288,
-1.08028414719823));
#82208=CARTESIAN_POINT('Ctrl Pts',(0.889133341739219,0.429979607970486,
-1.32320468901736));
#82209=CARTESIAN_POINT('Ctrl Pts',(0.968405565362423,1.34444024085867,-0.358362411303147));
#82210=CARTESIAN_POINT('Ctrl Pts',(1.04767778898562,1.03152012276366,0.933779522210948));
#82211=CARTESIAN_POINT('Ctrl Pts',(1.12695001260883,-0.223136159389758,
1.3733593350842));
#82212=CARTESIAN_POINT('Ctrl Pts',(1.20622223623203,-1.27407440626933,0.559170582466256));
#82213=CARTESIAN_POINT('Ctrl Pts',(1.28549445985523,-1.16185253682415,-0.765531104708832));
#82214=CARTESIAN_POINT('Ctrl Pts',(1.36476668347844,0.0110818382145732,
-1.39133265677073));
#82215=CARTESIAN_POINT('Ctrl Pts',(1.44403890710164,1.1738981497851,-0.746925431386865));
#82216=CARTESIAN_POINT('Ctrl Pts',(1.52331113072484,1.26500718194706,0.579388553442205));
#82217=CARTESIAN_POINT('Ctrl Pts',(1.60258335434805,0.201230401682631,1.37674954089208));
#82218=CARTESIAN_POINT('Ctrl Pts',(1.68185557797125,-1.04625910256907,0.917210803099231));
#82219=CARTESIAN_POINT('Ctrl Pts',(1.76112780159445,-1.33856870321064,-0.379693951816588));
#82220=CARTESIAN_POINT('Ctrl Pts',(1.84040002521766,-0.408834878719842,
-1.32995772423544));
#82221=CARTESIAN_POINT('Ctrl Pts',(1.91967224884086,0.894143840963125,-1.06603959552792));
#82222=CARTESIAN_POINT('Ctrl Pts',(1.99894447246406,1.3808158933056,0.17111712463292));
#82223=CARTESIAN_POINT('Ctrl Pts',(2.07821669608726,0.606875073722467,1.2520528059251));
#82224=CARTESIAN_POINT('Ctrl Pts',(2.15748891971047,-0.721111027024888,
1.18992961688625));
#82225=CARTESIAN_POINT('Ctrl Pts',(2.23676114333367,-1.39076037603547,0.0414627589559757));
#82226=CARTESIAN_POINT('Ctrl Pts',(2.31603336695688,-0.790718077312022,
-1.14485742507963));
#82227=CARTESIAN_POINT('Ctrl Pts',(2.39530559058008,0.53120860125257,-1.28598252302312));
#82228=CARTESIAN_POINT('Ctrl Pts',(2.47457781420328,1.36816948482281,-0.25307265184342));
#82229=CARTESIAN_POINT('Ctrl Pts',(2.55385003782648,0.956063119382725,1.01087931130145));
#82230=CARTESIAN_POINT('Ctrl Pts',(2.63312226144969,-0.328879200082413,
1.35195127086139));
#82231=CARTESIAN_POINT('Ctrl Pts',(2.71239448507289,-1.31357157456815,0.458762129424903));
#82232=CARTESIAN_POINT('Ctrl Pts',(2.7916667086961,-1.09904238472332,-0.853252660598941));
#82233=CARTESIAN_POINT('Ctrl Pts',(2.87093893231929,0.118856588721082,-1.38629274593749));
#82234=CARTESIAN_POINT('Ctrl Pts',(2.9502111559425,1.22824298214487,-0.653719011308979));
#82235=CARTESIAN_POINT('Ctrl Pts',(3.0294833795657,1.21631278230501,0.675664417594188));
#82236=CARTESIAN_POINT('Ctrl Pts',(3.10875560318891,0.0939426366750465,
1.38820463693965));
#82237=CARTESIAN_POINT('Ctrl Pts',(3.18802782681211,-1.11417351958857,0.833380451617229));
#82238=CARTESIAN_POINT('Ctrl Pts',(3.26730005043531,-1.30514299809352,-0.482265190838316));
#82239=CARTESIAN_POINT('Ctrl Pts',(3.34657227405852,-0.30451723605224,-1.35764959839504));
#82240=CARTESIAN_POINT('Ctrl Pts',(3.42584449768172,0.973987891872518,-0.993529415162783));
#82241=CARTESIAN_POINT('Ctrl Pts',(3.50511672130493,1.36353837168639,0.277552603562025));
#82242=CARTESIAN_POINT('Ctrl Pts',(3.58438894492812,0.507782087152296,1.29539343007532));
#82243=CARTESIAN_POINT('Ctrl Pts',(3.66366116855133,-0.810661450758132,
1.13032146536505));
#82244=CARTESIAN_POINT('Ctrl Pts',(3.74293339217452,-1.3907258022414,-0.0661218080816751));
#82245=CARTESIAN_POINT('Ctrl Pts',(3.82220561579774,-0.697731426064326,
-1.20332569137025));
#82246=CARTESIAN_POINT('Ctrl Pts',(3.87505376487987,0.183843906805461,-1.22728889992824));
#82247=CARTESIAN_POINT('Ctrl Pts',(3.90147783942094,0.532641718062236,-1.05042270666609));
#82248=CARTESIAN_POINT('Ctrl Pts',(3.7365,0.66187319412785,-1.30528009442227));
#82249=CARTESIAN_POINT('Ctrl Pts',(3.71007592545893,0.228448785913637,-1.5250582084865));
#82250=CARTESIAN_POINT('Ctrl Pts',(3.68365185091787,-0.319284391609157,
-1.51016958368301));
#82251=CARTESIAN_POINT('Ctrl Pts',(3.6572277763768,-0.736672846858221,-1.26720586518308));
#82252=CARTESIAN_POINT('Ctrl Pts',(3.63080370183573,-1.15406130210729,-1.02424214668315));
#82253=CARTESIAN_POINT('Ctrl Pts',(3.60437962729466,-1.44110503508263,-0.553203334486778));
#82254=CARTESIAN_POINT('Ctrl Pts',(3.5779555527536,-1.46449328826871,-0.0698958111184731));
#82255=CARTESIAN_POINT('Ctrl Pts',(3.5766887171167,-1.46561457910426,-0.0467248503632885));
#82256=CARTESIAN_POINT('Ctrl Pts',(3.5754218814798,-1.46612986275361,-0.0235256902050746));
#82257=CARTESIAN_POINT('Ctrl Pts',(3.57415504584291,-1.46605134156425,-0.000323220338867419));
#82258=CARTESIAN_POINT('Origin',(4.,0.,0.866025403784439));
#82259=CARTESIAN_POINT('',(4.,5.30287619362453E-17,0.866025403784439));
#82260=CARTESIAN_POINT('',(4.,0.75,0.433012701892219));
#82261=CARTESIAN_POINT('',(4.,0.1875,0.757772228311384));
#82262=CARTESIAN_POINT('',(2.,0.,0.866025403784439));
#82263=CARTESIAN_POINT('',(4.,5.30287619362453E-17,0.866025403784439));
#82264=CARTESIAN_POINT('',(2.,0.75,0.433012701892219));
#82265=CARTESIAN_POINT('',(2.,0.75,0.433012701892219));
#82266=CARTESIAN_POINT('',(4.,0.75,0.433012701892219));
#82267=CARTESIAN_POINT('Origin',(4.,-0.75,0.433012701892219));
#82268=CARTESIAN_POINT('',(4.,-0.75,0.433012701892219));
#82269=CARTESIAN_POINT('',(4.,-0.5625,0.541265877365274));
#82270=CARTESIAN_POINT('',(2.,-0.75,0.433012701892219));
#82271=CARTESIAN_POINT('',(4.,-0.75,0.433012701892219));
#82272=CARTESIAN_POINT('',(2.,5.30287619362453E-17,0.866025403784439));
#82273=CARTESIAN_POINT('Origin',(4.,-0.75,-0.433012701892219));
#82274=CARTESIAN_POINT('',(4.,-0.75,-0.433012701892219));
#82275=CARTESIAN_POINT('',(4.,-0.75,-0.21650635094611));
#82276=CARTESIAN_POINT('',(2.,-0.75,-0.433012701892219));
#82277=CARTESIAN_POINT('',(4.,-0.75,-0.433012701892219));
#82278=CARTESIAN_POINT('',(2.,-0.75,0.433012701892219));
#82279=CARTESIAN_POINT('Origin',(4.,-1.38777878078145E-16,-0.866025403784439));
#82280=CARTESIAN_POINT('',(4.,-1.59086285808736E-16,-0.866025403784439));
#82281=CARTESIAN_POINT('',(4.,-0.1875,-0.757772228311384));
#82282=CARTESIAN_POINT('',(2.,-1.38777878078145E-16,-0.866025403784439));
#82283=CARTESIAN_POINT('',(4.,-1.59086285808736E-16,-0.866025403784439));
#82284=CARTESIAN_POINT('',(2.,-0.75,-0.433012701892219));
#82285=CARTESIAN_POINT('Origin',(4.,0.75,-0.43301270189222));
#82286=CARTESIAN_POINT('',(4.,0.75,-0.43301270189222));
#82287=CARTESIAN_POINT('',(4.,0.5625,-0.541265877365275));
#82288=CARTESIAN_POINT('',(2.,0.75,-0.43301270189222));
#82289=CARTESIAN_POINT('',(4.,0.75,-0.43301270189222));
#82290=CARTESIAN_POINT('',(2.,-1.59086285808736E-16,-0.866025403784439));
#82291=CARTESIAN_POINT('Origin',(4.,0.75,0.433012701892219));
#82292=CARTESIAN_POINT('',(4.,0.75,0.21650635094611));
#82293=CARTESIAN_POINT('',(2.,0.75,-0.43301270189222));
#82294=CARTESIAN_POINT('Origin',(2.,0.,0.));
#82295=CARTESIAN_POINT('Origin',(0.,1.05,0.));
#82296=CARTESIAN_POINT('',(0.,-1.05,-1.28587913910472E-16));
#82297=CARTESIAN_POINT('Origin',(0.,0.,0.));
#82298=CARTESIAN_POINT('Origin',(0.225,0.,0.));
#82299=CARTESIAN_POINT('',(0.225,-1.275,-1.56142466891288E-16));
#82300=CARTESIAN_POINT('Origin',(2.075,0.,0.));
#82301=CARTESIAN_POINT('Origin',(3.7365,0.,0.));
#82302=CARTESIAN_POINT('Origin',(3.85,0.,0.));
#82303=CARTESIAN_POINT('',(4.,-1.2,-1.46957615897682E-16));
#82304=CARTESIAN_POINT('Origin',(4.,0.,0.));
#82305=CARTESIAN_POINT('',(3.85,-1.35,-1.65327317884893E-16));
#82306=CARTESIAN_POINT('Origin',(4.,0.,0.));
#82362=UNCERTAINTY_MEASURE_WITH_UNIT(LENGTH_MEASURE(0.01),#82385,
'DISTANCE_ACCURACY_VALUE',
'Maximum model space distance between geometric entities at asserted c
onnectivities');
#82363=UNCERTAINTY_MEASURE_WITH_UNIT(LENGTH_MEASURE(0.01),#82385,
'DISTANCE_ACCURACY_VALUE',
'Maximum model space distance between geometric entities at asserted c
onnectivities');
#82383=(
GEOMETRIC_REPRESENTATION_CONTEXT(3)
GLOBAL_UNCERTAINTY_ASSIGNED_CONTEXT((#82362))
GLOBAL_UNIT_ASSIGNED_CONTEXT((#82385,#82387,#82388))
REPRESENTATION_CONTEXT('','3D')
);
#82384=(
GEOMETRIC_REPRESENTATION_CONTEXT(3)
GLOBAL_UNCERTAINTY_ASSIGNED_CONTEXT((#82363))
GLOBAL_UNIT_ASSIGNED_CONTEXT((#82385,#82387,#82388))
REPRESENTATION_CONTEXT('','3D')
);
#82385=(
LENGTH_UNIT()
NAMED_UNIT(*)
SI_UNIT(.MILLI.,.METRE.)
);
#82387=(
NAMED_UNIT(*)
PLANE_ANGLE_UNIT()
SI_UNIT($,.RADIAN.)
);
#82388=(
NAMED_UNIT(*)
SI_UNIT($,.STERADIAN.)
SOLID_ANGLE_UNIT()
);
#82408=SHAPE_DEFINITION_REPRESENTATION(#82428,#82484);
#82428=PRODUCT_DEFINITION_SHAPE('',$,#82505);
#82484=SHAPE_REPRESENTATION('',(#33338),#82383);
#82485=PRODUCT_DEFINITION_CONTEXT('part definition',#82547,'design');
#82505=PRODUCT_DEFINITION('2026-10-20-12-38-42-004',
'19_ISO_4026_Set_Screw_M3x4',#82525,#82485);
#82525=PRODUCT_DEFINITION_FORMATION('',$,#82568);
#82547=APPLICATION_CONTEXT(
'Core Data for Automotive Mechanical Design Process');
#82548=PRODUCT_CONTEXT('part definition',#82547,'mechanical');
#82568=PRODUCT('2026-10-20-12-38-42-004','19_ISO_4026_Set_Screw_M3x4',$,
(#82548));
#82632=COLOUR_RGB('Black',0.12,0.14,0.17);
#82633=FILL_AREA_STYLE_COLOUR('',#82632);
#82634=FILL_AREA_STYLE('',(#82633));
#82635=SURFACE_STYLE_FILL_AREA(#82634);
#82636=SURFACE_SIDE_STYLE('',(#82635));
#82637=SURFACE_STYLE_USAGE(.BOTH.,#82636);
#82638=PRESENTATION_STYLE_ASSIGNMENT((#82637));
ENDSEC;
END-ISO-10303-21;
